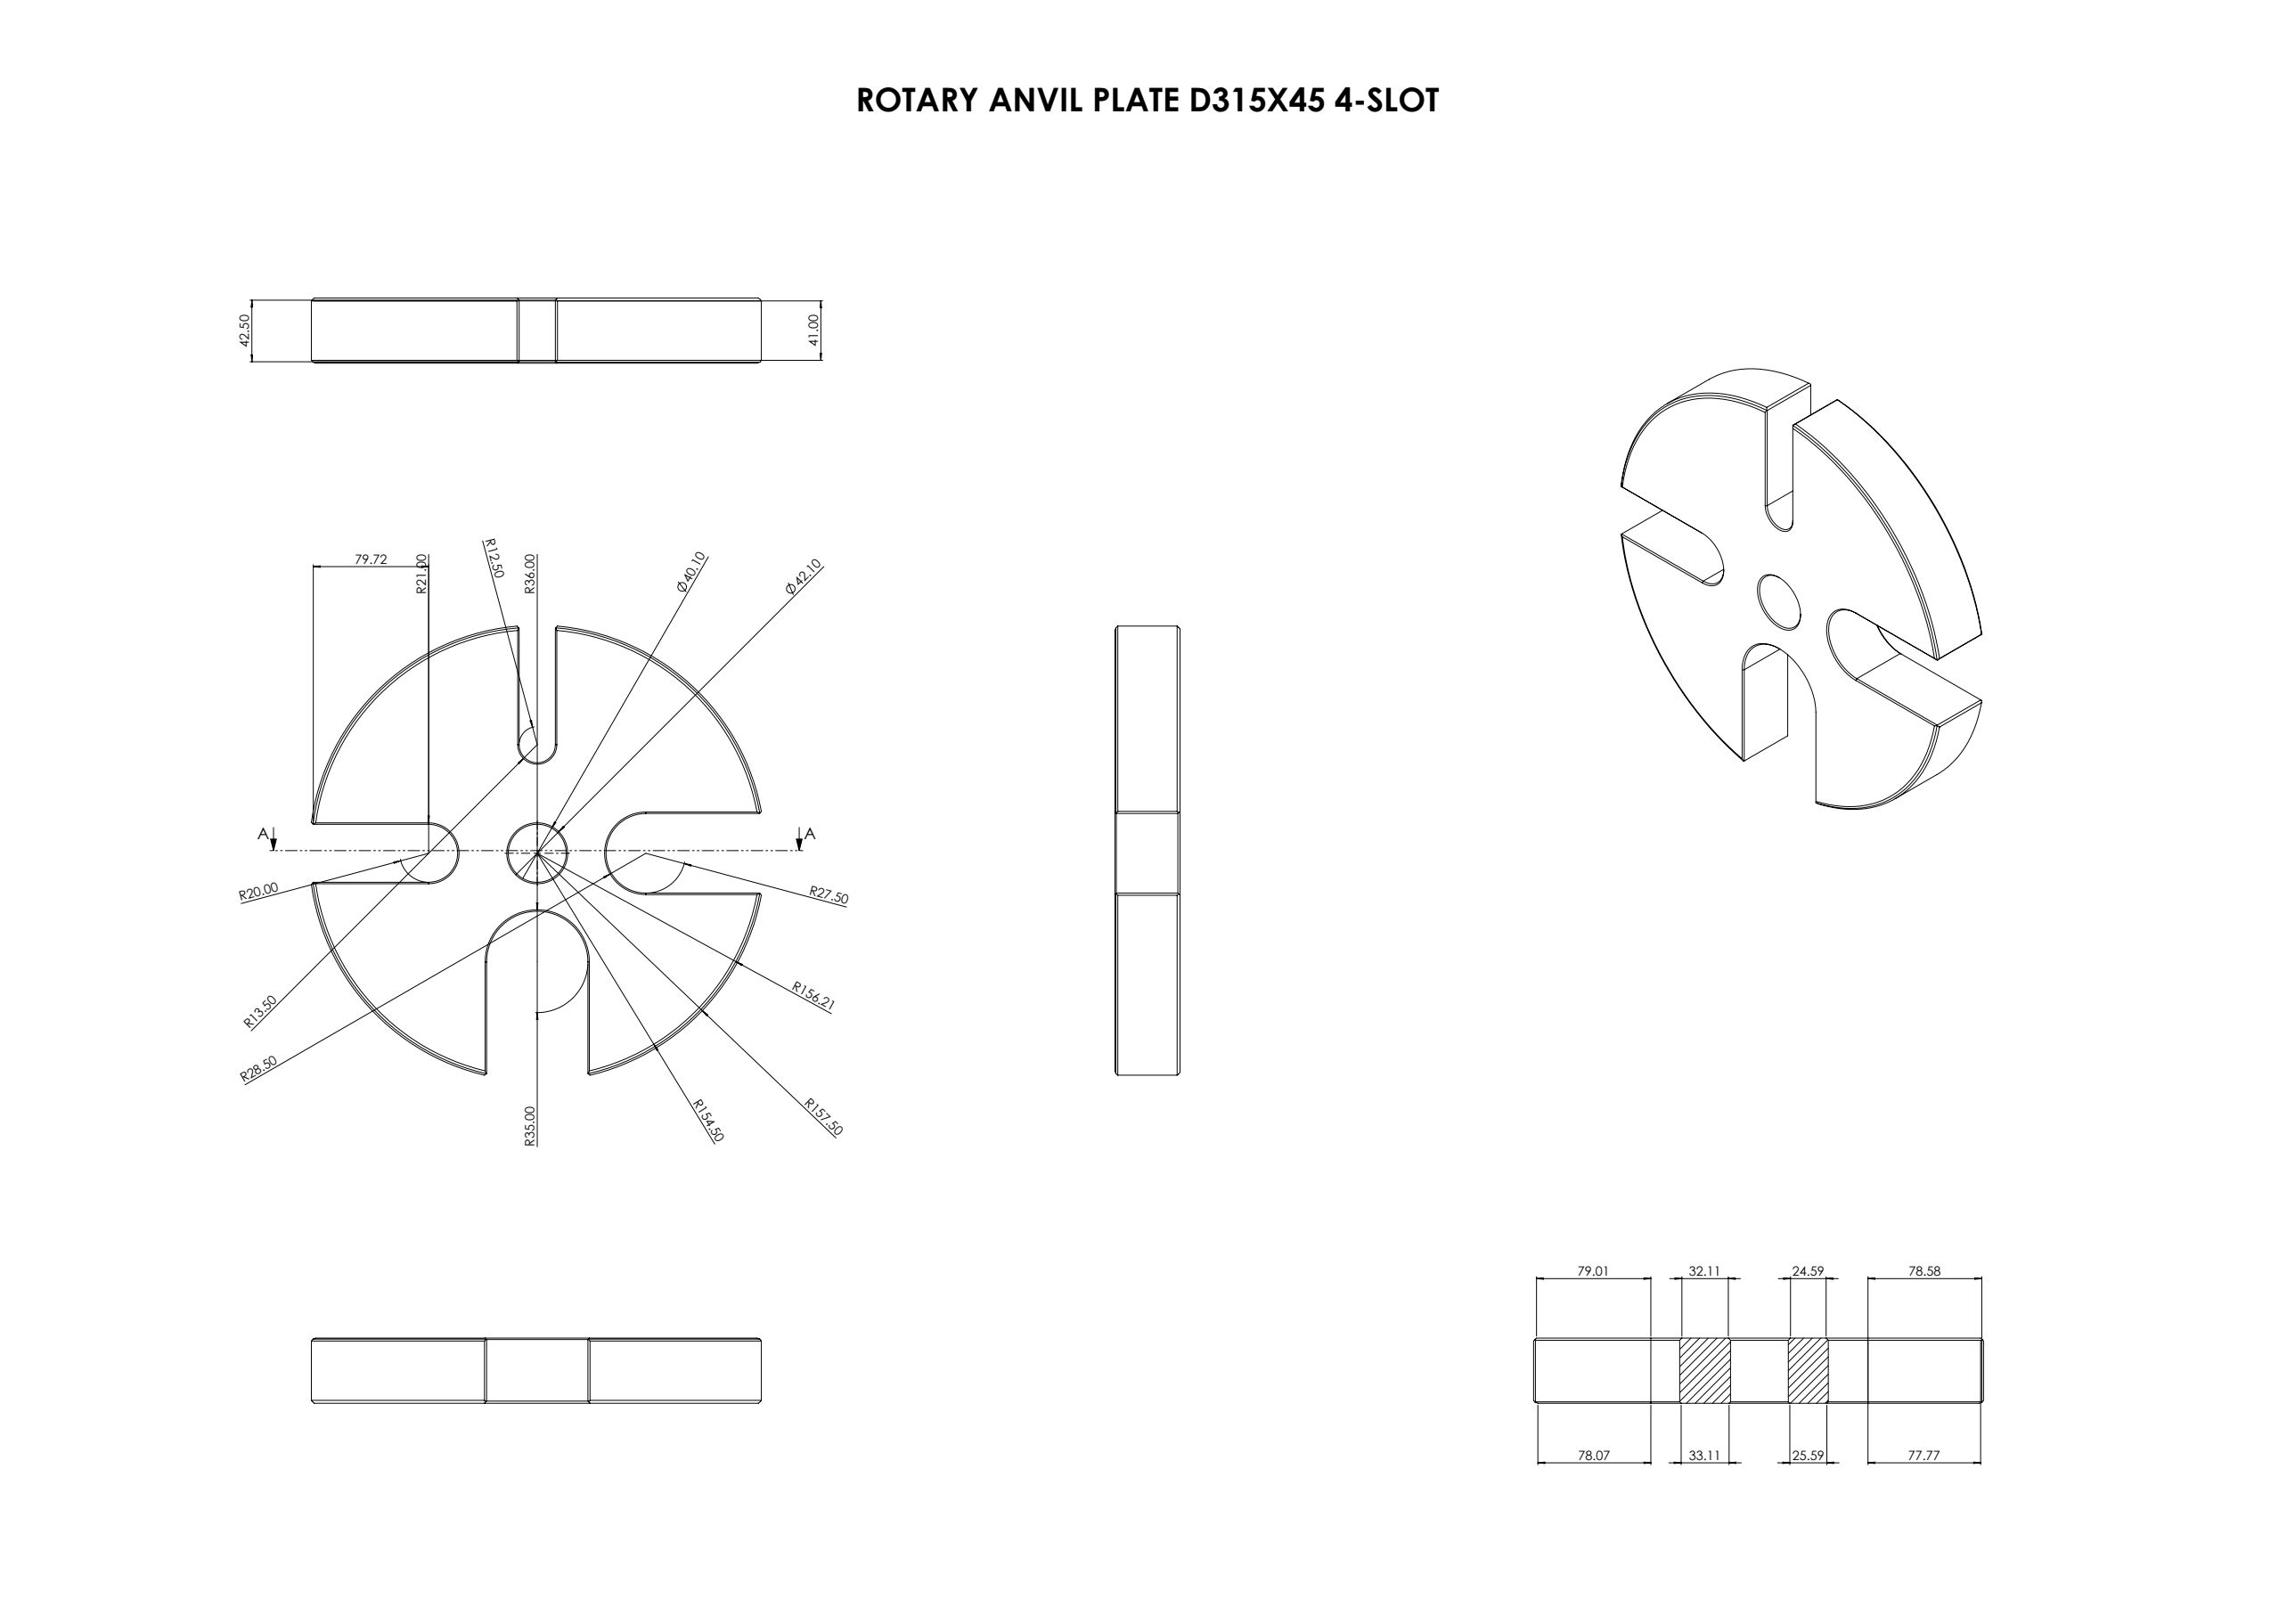
ISO-10303-21;
HEADER;
/* Generated by software containing ST-Developer
 * from STEP Tools, Inc. (www.steptools.com) 
 */

FILE_DESCRIPTION(
/* description */ (''),
/* implementation_level */ '2;1');

FILE_NAME(
/* name */ '08_Rotary_Anvil_Plate_D315x45_4-Slot.step',
/* time_stamp */ '2026-10-19T23:58:09-07:00',
/* author */ (''),
/* organization */ (''),
/* preprocessor_version */ 'ST-DEVELOPER v20.2',
/* originating_system */ 'Autodesk Translation Framework v15.15.0.0',
/* authorisation */ '');

FILE_SCHEMA (('AP203_CONFIGURATION_CONTROLLED_3D_DESIGN_OF_MECHANICAL_PARTS_AND_ASSEMBLIES_MIM_LF { 1 0 10303 203 3 1 4 }',
'AUTOMOTIVE_DESIGN { 1 0 10303 214 3 1 1 }','INTEGRATED_CNC_SCHEMA','MODEL_BASED_INTEGRATED_MANUFACTURING_SCHEMA',
'PROCESS_PLANNING_SCHEMA','AP242_MANAGED_MODEL_BASED_3D_ENGINEERING_MIM_LF { 1 0 10303 442 3 1 4 }'));
ENDSEC;

DATA;
#10=MECHANICAL_DESIGN_GEOMETRIC_PRESENTATION_REPRESENTATION('',(#409),#70757);
#171=(
BOUNDED_CURVE()
B_SPLINE_CURVE(2,(#43625,#43626,#43627),.UNSPECIFIED.,.F.,.F.)
B_SPLINE_CURVE_WITH_KNOTS((3,3),(0.00762589341662222,0.217939135937014),
 .UNSPECIFIED.)
CURVE()
GEOMETRIC_REPRESENTATION_ITEM()
RATIONAL_B_SPLINE_CURVE((1.00000105618797,1.00001509230994,1.))
REPRESENTATION_ITEM('')
);
#172=(
BOUNDED_CURVE()
B_SPLINE_CURVE(2,(#43631,#43632,#43633),.UNSPECIFIED.,.F.,.F.)
B_SPLINE_CURVE_WITH_KNOTS((3,3),(0.,0.167475634560782),.UNSPECIFIED.)
CURVE()
GEOMETRIC_REPRESENTATION_ITEM()
RATIONAL_B_SPLINE_CURVE((1.,1.00001872457605,1.00001886903166))
REPRESENTATION_ITEM('')
);
#173=(
BOUNDED_CURVE()
B_SPLINE_CURVE(2,(#43647,#43648,#43649),.UNSPECIFIED.,.F.,.F.)
B_SPLINE_CURVE_WITH_KNOTS((3,3),(0.137287012047938,0.14598329580768),
 .UNSPECIFIED.)
CURVE()
GEOMETRIC_REPRESENTATION_ITEM()
RATIONAL_B_SPLINE_CURVE((1.,1.,1.))
REPRESENTATION_ITEM('')
);
#174=(
BOUNDED_CURVE()
B_SPLINE_CURVE(2,(#43653,#43654,#43655),.UNSPECIFIED.,.F.,.F.)
B_SPLINE_CURVE_WITH_KNOTS((3,3),(7.75867498909367,7.76962220124035),
 .UNSPECIFIED.)
CURVE()
GEOMETRIC_REPRESENTATION_ITEM()
RATIONAL_B_SPLINE_CURVE((1.,1.,1.))
REPRESENTATION_ITEM('')
);
#175=(
BOUNDED_CURVE()
B_SPLINE_CURVE(2,(#43656,#43657,#43658),.UNSPECIFIED.,.F.,.F.)
B_SPLINE_CURVE_WITH_KNOTS((3,3),(0.,0.20316916463777),.UNSPECIFIED.)
CURVE()
GEOMETRIC_REPRESENTATION_ITEM()
RATIONAL_B_SPLINE_CURVE((1.,1.00001376388279,1.00000116347276))
REPRESENTATION_ITEM('')
);
#176=(
BOUNDED_CURVE()
B_SPLINE_CURVE(2,(#43673,#43674,#43675),.UNSPECIFIED.,.F.,.F.)
B_SPLINE_CURVE_WITH_KNOTS((3,3),(0.170079793729576,0.3375554282914),
 .UNSPECIFIED.)
CURVE()
GEOMETRIC_REPRESENTATION_ITEM()
RATIONAL_B_SPLINE_CURVE((1.00001886905196,1.00001872459619,1.))
REPRESENTATION_ITEM('')
);
#177=(
BOUNDED_CURVE()
B_SPLINE_CURVE(2,(#43679,#43680,#43681),.UNSPECIFIED.,.F.,.F.)
B_SPLINE_CURVE_WITH_KNOTS((3,3),(0.,0.210313242519936),.UNSPECIFIED.)
CURVE()
GEOMETRIC_REPRESENTATION_ITEM()
RATIONAL_B_SPLINE_CURVE((1.,1.00001509226017,1.00000105618449))
REPRESENTATION_ITEM('')
);
#178=(
BOUNDED_CURVE()
B_SPLINE_CURVE(2,(#43694,#43695,#43696),.UNSPECIFIED.,.F.,.F.)
B_SPLINE_CURVE_WITH_KNOTS((3,3),(0.,0.17930472101048),.UNSPECIFIED.)
CURVE()
GEOMETRIC_REPRESENTATION_ITEM()
RATIONAL_B_SPLINE_CURVE((1.,1.,1.))
REPRESENTATION_ITEM('')
);
#179=(
BOUNDED_CURVE()
B_SPLINE_CURVE(2,(#43703,#43704,#43705),.UNSPECIFIED.,.F.,.F.)
B_SPLINE_CURVE_WITH_KNOTS((3,3),(7.54305180428147,7.55174808804129),
 .UNSPECIFIED.)
CURVE()
GEOMETRIC_REPRESENTATION_ITEM()
RATIONAL_B_SPLINE_CURVE((1.,1.,1.))
REPRESENTATION_ITEM('')
);
#180=(
BOUNDED_CURVE()
B_SPLINE_CURVE(2,(#43722,#43723,#43724),.UNSPECIFIED.,.F.,.F.)
B_SPLINE_CURVE_WITH_KNOTS((3,3),(0.177416517606212,0.356721238616782),
 .UNSPECIFIED.)
CURVE()
GEOMETRIC_REPRESENTATION_ITEM()
RATIONAL_B_SPLINE_CURVE((1.,1.,1.))
REPRESENTATION_ITEM('')
);
#181=(
BOUNDED_CURVE()
B_SPLINE_CURVE(2,(#43757,#43758,#43759),.UNSPECIFIED.,.F.,.F.)
B_SPLINE_CURVE_WITH_KNOTS((3,3),(0.166982558562854,0.32848249154248),
 .UNSPECIFIED.)
CURVE()
GEOMETRIC_REPRESENTATION_ITEM()
RATIONAL_B_SPLINE_CURVE((1.00001732315097,1.00001703876093,1.))
REPRESENTATION_ITEM('')
);
#182=(
BOUNDED_CURVE()
B_SPLINE_CURVE(2,(#43760,#43761,#43762),.UNSPECIFIED.,.F.,.F.)
B_SPLINE_CURVE_WITH_KNOTS((3,3),(0.,0.188171618307079),.UNSPECIFIED.)
CURVE()
GEOMETRIC_REPRESENTATION_ITEM()
RATIONAL_B_SPLINE_CURVE((1.,1.,1.))
REPRESENTATION_ITEM('')
);
#183=(
BOUNDED_CURVE()
B_SPLINE_CURVE(2,(#43766,#43767,#43768),.UNSPECIFIED.,.F.,.F.)
B_SPLINE_CURVE_WITH_KNOTS((3,3),(0.00896598248719952,0.212135147124771),
 .UNSPECIFIED.)
CURVE()
GEOMETRIC_REPRESENTATION_ITEM()
RATIONAL_B_SPLINE_CURVE((1.00000116347024,1.00001376385308,1.))
REPRESENTATION_ITEM('')
);
#184=(
BOUNDED_CURVE()
B_SPLINE_CURVE(2,(#43772,#43773,#43774),.UNSPECIFIED.,.F.,.F.)
B_SPLINE_CURVE_WITH_KNOTS((3,3),(0.,0.161499932979635),.UNSPECIFIED.)
CURVE()
GEOMETRIC_REPRESENTATION_ITEM()
RATIONAL_B_SPLINE_CURVE((1.,1.00001703876093,1.00001732315097))
REPRESENTATION_ITEM('')
);
#185=(
BOUNDED_CURVE()
B_SPLINE_CURVE(2,(#43792,#43793,#43794),.UNSPECIFIED.,.F.,.F.)
B_SPLINE_CURVE_WITH_KNOTS((3,3),(0.143033593949376,0.153980806095915),
 .UNSPECIFIED.)
CURVE()
GEOMETRIC_REPRESENTATION_ITEM()
RATIONAL_B_SPLINE_CURVE((1.,1.,1.))
REPRESENTATION_ITEM('')
);
#186=(
BOUNDED_CURVE()
B_SPLINE_CURVE(2,(#43800,#43801,#43802),.UNSPECIFIED.,.F.,.F.)
B_SPLINE_CURVE_WITH_KNOTS((3,3),(0.18255185197649,0.370723470283569),
 .UNSPECIFIED.)
CURVE()
GEOMETRIC_REPRESENTATION_ITEM()
RATIONAL_B_SPLINE_CURVE((1.,1.,1.))
REPRESENTATION_ITEM('')
);
#187=(
BOUNDED_CURVE()
B_SPLINE_CURVE(2,(#43820,#43821,#43822),.UNSPECIFIED.,.F.,.F.)
B_SPLINE_CURVE_WITH_KNOTS((3,3),(0.166073953914202,0.324403911055146),
 .UNSPECIFIED.)
CURVE()
GEOMETRIC_REPRESENTATION_ITEM()
RATIONAL_B_SPLINE_CURVE((1.00001663891698,1.00001625098222,1.))
REPRESENTATION_ITEM('')
);
#188=(
BOUNDED_CURVE()
B_SPLINE_CURVE(2,(#43823,#43824,#43825),.UNSPECIFIED.,.F.,.F.)
B_SPLINE_CURVE_WITH_KNOTS((3,3),(0.,0.193708051007078),.UNSPECIFIED.)
CURVE()
GEOMETRIC_REPRESENTATION_ITEM()
RATIONAL_B_SPLINE_CURVE((1.,1.,1.))
REPRESENTATION_ITEM('')
);
#189=(
BOUNDED_CURVE()
B_SPLINE_CURVE(2,(#43843,#43844,#43845),.UNSPECIFIED.,.F.,.F.)
B_SPLINE_CURVE_WITH_KNOTS((3,3),(0.00815575297236999,0.214933042676883),
 .UNSPECIFIED.)
CURVE()
GEOMETRIC_REPRESENTATION_ITEM()
RATIONAL_B_SPLINE_CURVE((1.00000109358995,1.00001440998863,1.))
REPRESENTATION_ITEM('')
);
#190=(
BOUNDED_CURVE()
B_SPLINE_CURVE(2,(#43849,#43850,#43851),.UNSPECIFIED.,.F.,.F.)
B_SPLINE_CURVE_WITH_KNOTS((3,3),(0.,0.164543974719834),.UNSPECIFIED.)
CURVE()
GEOMETRIC_REPRESENTATION_ITEM()
RATIONAL_B_SPLINE_CURVE((1.,1.00001786148183,1.00001806362432))
REPRESENTATION_ITEM('')
);
#191=(
BOUNDED_CURVE()
B_SPLINE_CURVE(2,(#43869,#43870,#43871),.UNSPECIFIED.,.F.,.F.)
B_SPLINE_CURVE_WITH_KNOTS((3,3),(0.140031413282733,0.149652192224334),
 .UNSPECIFIED.)
CURVE()
GEOMETRIC_REPRESENTATION_ITEM()
RATIONAL_B_SPLINE_CURVE((1.,1.,1.))
REPRESENTATION_ITEM('')
);
#192=(
BOUNDED_CURVE()
B_SPLINE_CURVE(2,(#43877,#43878,#43879),.UNSPECIFIED.,.F.,.F.)
B_SPLINE_CURVE_WITH_KNOTS((3,3),(0.180004690478429,0.363403446267975),
 .UNSPECIFIED.)
CURVE()
GEOMETRIC_REPRESENTATION_ITEM()
RATIONAL_B_SPLINE_CURVE((1.,1.,1.))
REPRESENTATION_ITEM('')
);
#193=(
BOUNDED_CURVE()
B_SPLINE_CURVE(2,(#43884,#43885,#43886),.UNSPECIFIED.,.F.,.F.)
B_SPLINE_CURVE_WITH_KNOTS((3,3),(0.168310970500792,0.332854945221182),
 .UNSPECIFIED.)
CURVE()
GEOMETRIC_REPRESENTATION_ITEM()
RATIONAL_B_SPLINE_CURVE((1.00001806363053,1.00001786148798,1.))
REPRESENTATION_ITEM('')
);
#194=(
BOUNDED_CURVE()
B_SPLINE_CURVE(2,(#43890,#43891,#43892),.UNSPECIFIED.,.F.,.F.)
B_SPLINE_CURVE_WITH_KNOTS((3,3),(0.,0.206777289704965),.UNSPECIFIED.)
CURVE()
GEOMETRIC_REPRESENTATION_ITEM()
RATIONAL_B_SPLINE_CURVE((1.,1.00001441002009,1.00000109359234))
REPRESENTATION_ITEM('')
);
#195=(
BOUNDED_CURVE()
B_SPLINE_CURVE(2,(#43905,#43906,#43907),.UNSPECIFIED.,.F.,.F.)
B_SPLINE_CURVE_WITH_KNOTS((3,3),(0.,0.183398755789119),.UNSPECIFIED.)
CURVE()
GEOMETRIC_REPRESENTATION_ITEM()
RATIONAL_B_SPLINE_CURVE((1.,1.,1.))
REPRESENTATION_ITEM('')
);
#196=(
BOUNDED_CURVE()
B_SPLINE_CURVE(2,(#43909,#43910,#43911),.UNSPECIFIED.,.F.,.F.)
B_SPLINE_CURVE_WITH_KNOTS((3,3),(0.185074227573043,0.378782278580072),
 .UNSPECIFIED.)
CURVE()
GEOMETRIC_REPRESENTATION_ITEM()
RATIONAL_B_SPLINE_CURVE((1.,1.,1.))
REPRESENTATION_ITEM('')
);
#197=(
BOUNDED_CURVE()
B_SPLINE_CURVE(2,(#43912,#43913,#43914),.UNSPECIFIED.,.F.,.F.)
B_SPLINE_CURVE_WITH_KNOTS((3,3),(0.,0.158329957141101),.UNSPECIFIED.)
CURVE()
GEOMETRIC_REPRESENTATION_ITEM()
RATIONAL_B_SPLINE_CURVE((1.,1.00001625097861,1.00001663891328))
REPRESENTATION_ITEM('')
);
#198=(
BOUNDED_CURVE()
B_SPLINE_CURVE(2,(#43929,#43930,#43931),.UNSPECIFIED.,.F.,.F.)
B_SPLINE_CURVE_WITH_KNOTS((3,3),(0.0100528190707853,0.209523932952566),
 .UNSPECIFIED.)
CURVE()
GEOMETRIC_REPRESENTATION_ITEM()
RATIONAL_B_SPLINE_CURVE((1.00000126177961,1.00001314919847,1.))
REPRESENTATION_ITEM('')
);
#199=(
BOUNDED_CURVE()
B_SPLINE_CURVE(2,(#43949,#43950,#43951),.UNSPECIFIED.,.F.,.F.)
B_SPLINE_CURVE_WITH_KNOTS((3,3),(0.146334104657409,0.159049105721225),
 .UNSPECIFIED.)
CURVE()
GEOMETRIC_REPRESENTATION_ITEM()
RATIONAL_B_SPLINE_CURVE((1.,1.,1.))
REPRESENTATION_ITEM('')
);
#200=(
BOUNDED_CURVE()
B_SPLINE_CURVE(2,(#43962,#43963,#43964),.UNSPECIFIED.,.F.,.F.)
B_SPLINE_CURVE_WITH_KNOTS((3,3),(0.,0.199471113881606),.UNSPECIFIED.)
CURVE()
GEOMETRIC_REPRESENTATION_ITEM()
RATIONAL_B_SPLINE_CURVE((1.,1.00001314920547,1.00000126178028))
REPRESENTATION_ITEM('')
);
#201=(
BOUNDED_CURVE()
B_SPLINE_CURVE(2,(#44023,#44024,#44025),.UNSPECIFIED.,.F.,.F.)
B_SPLINE_CURVE_WITH_KNOTS((3,3),(7.87870547859755,7.89142047966152),
 .UNSPECIFIED.)
CURVE()
GEOMETRIC_REPRESENTATION_ITEM()
RATIONAL_B_SPLINE_CURVE((1.,1.,1.))
REPRESENTATION_ITEM('')
);
#202=(
BOUNDED_CURVE()
B_SPLINE_CURVE(2,(#44035,#44036,#44037),.UNSPECIFIED.,.F.,.F.)
B_SPLINE_CURVE_WITH_KNOTS((3,3),(7.6471088967316,7.6567296756733),
 .UNSPECIFIED.)
CURVE()
GEOMETRIC_REPRESENTATION_ITEM()
RATIONAL_B_SPLINE_CURVE((1.,1.,1.))
REPRESENTATION_ITEM('')
);
#379=SHAPE_REPRESENTATION_RELATIONSHIP('SRR','None',#70820,#394);
#394=ADVANCED_BREP_SHAPE_REPRESENTATION('',(#469),#70744);
#409=STYLED_ITEM('',(#71033),#469);
#469=MANIFOLD_SOLID_BREP('Anvil',#26874);
#587=CYLINDRICAL_SURFACE('',#27285,15.75);
#588=CYLINDRICAL_SURFACE('',#27319,2.75);
#589=CYLINDRICAL_SURFACE('',#27324,2.005);
#590=CYLINDRICAL_SURFACE('',#27331,15.75);
#591=CYLINDRICAL_SURFACE('',#27338,2.);
#592=CYLINDRICAL_SURFACE('',#27346,15.75);
#593=CYLINDRICAL_SURFACE('',#27351,3.5);
#594=CYLINDRICAL_SURFACE('',#27382,1.25);
#595=CYLINDRICAL_SURFACE('',#27386,15.75);
#850=FACE_BOUND('',#4238,.T.);
#851=FACE_BOUND('',#4287,.T.);
#1094=B_SPLINE_CURVE_WITH_KNOTS('',3,(#43666,#43667,#43668,#43669),
 .UNSPECIFIED.,.F.,.F.,(4,4),(0.,0.203579345120206),.UNSPECIFIED.);
#1095=B_SPLINE_CURVE_WITH_KNOTS('',3,(#43707,#43708,#43709,#43710),
 .UNSPECIFIED.,.F.,.F.,(4,4),(0.,0.203579415270987),.UNSPECIFIED.);
#1096=B_SPLINE_CURVE_WITH_KNOTS('',3,(#43788,#43789,#43790,#43791),
 .UNSPECIFIED.,.F.,.F.,(4,4),(0.,0.211711806319391),.UNSPECIFIED.);
#1097=B_SPLINE_CURVE_WITH_KNOTS('',3,(#43865,#43866,#43867,#43868),
 .UNSPECIFIED.,.F.,.F.,(4,4),(0.,0.207414265317584),.UNSPECIFIED.);
#1098=B_SPLINE_CURVE_WITH_KNOTS('',3,(#43945,#43946,#43947,#43948),
 .UNSPECIFIED.,.F.,.F.,(4,4),(0.,0.21653079565574),.UNSPECIFIED.);
#1099=B_SPLINE_CURVE_WITH_KNOTS('',3,(#43992,#43993,#43994,#43995),
 .UNSPECIFIED.,.F.,.F.,(4,4),(0.,0.207414336599568),.UNSPECIFIED.);
#1100=B_SPLINE_CURVE_WITH_KNOTS('',3,(#43999,#44000,#44001,#44002),
 .UNSPECIFIED.,.F.,.F.,(4,4),(0.,0.211711879270631),.UNSPECIFIED.);
#1101=B_SPLINE_CURVE_WITH_KNOTS('',3,(#44008,#44009,#44010,#44011),
 .UNSPECIFIED.,.F.,.F.,(4,4),(0.,0.216530870858263),.UNSPECIFIED.);
#1727=PLANE('',#27284);
#1728=PLANE('',#27290);
#1729=PLANE('',#27291);
#1730=PLANE('',#27292);
#1731=PLANE('',#27293);
#1732=PLANE('',#27294);
#1733=PLANE('',#27298);
#1734=PLANE('',#27299);
#1735=PLANE('',#27309);
#1736=PLANE('',#27310);
#1737=PLANE('',#27311);
#1738=PLANE('',#27312);
#1739=PLANE('',#27313);
#1740=PLANE('',#27314);
#1741=PLANE('',#27321);
#1742=PLANE('',#27326);
#1743=PLANE('',#27327);
#1744=PLANE('',#27328);
#1745=PLANE('',#27329);
#1746=PLANE('',#27330);
#1747=PLANE('',#27335);
#1748=PLANE('',#27340);
#1749=PLANE('',#27341);
#1750=PLANE('',#27342);
#1751=PLANE('',#27343);
#1752=PLANE('',#27344);
#1753=PLANE('',#27345);
#1754=PLANE('',#27348);
#1755=PLANE('',#27353);
#1756=PLANE('',#27367);
#1757=PLANE('',#27370);
#1758=PLANE('',#27376);
#1759=PLANE('',#27379);
#1760=PLANE('',#27383);
#2733=FACE_OUTER_BOUND('',#4227,.T.);
#2734=FACE_OUTER_BOUND('',#4228,.T.);
#2735=FACE_OUTER_BOUND('',#4229,.T.);
#2736=FACE_OUTER_BOUND('',#4230,.T.);
#2737=FACE_OUTER_BOUND('',#4231,.T.);
#2738=FACE_OUTER_BOUND('',#4232,.T.);
#2739=FACE_OUTER_BOUND('',#4233,.T.);
#2740=FACE_OUTER_BOUND('',#4234,.T.);
#2741=FACE_OUTER_BOUND('',#4235,.T.);
#2742=FACE_OUTER_BOUND('',#4236,.T.);
#2743=FACE_OUTER_BOUND('',#4237,.T.);
#2744=FACE_OUTER_BOUND('',#4239,.T.);
#2745=FACE_OUTER_BOUND('',#4240,.T.);
#2746=FACE_OUTER_BOUND('',#4241,.T.);
#2747=FACE_OUTER_BOUND('',#4242,.T.);
#2748=FACE_OUTER_BOUND('',#4243,.T.);
#2749=FACE_OUTER_BOUND('',#4244,.T.);
#2750=FACE_OUTER_BOUND('',#4245,.T.);
#2751=FACE_OUTER_BOUND('',#4246,.T.);
#2752=FACE_OUTER_BOUND('',#4247,.T.);
#2753=FACE_OUTER_BOUND('',#4248,.T.);
#2754=FACE_OUTER_BOUND('',#4249,.T.);
#2755=FACE_OUTER_BOUND('',#4250,.T.);
#2756=FACE_OUTER_BOUND('',#4251,.T.);
#2757=FACE_OUTER_BOUND('',#4252,.T.);
#2758=FACE_OUTER_BOUND('',#4253,.T.);
#2759=FACE_OUTER_BOUND('',#4254,.T.);
#2760=FACE_OUTER_BOUND('',#4255,.T.);
#2761=FACE_OUTER_BOUND('',#4256,.T.);
#2762=FACE_OUTER_BOUND('',#4257,.T.);
#2763=FACE_OUTER_BOUND('',#4258,.T.);
#2764=FACE_OUTER_BOUND('',#4259,.T.);
#2765=FACE_OUTER_BOUND('',#4260,.T.);
#2766=FACE_OUTER_BOUND('',#4261,.T.);
#2767=FACE_OUTER_BOUND('',#4262,.T.);
#2768=FACE_OUTER_BOUND('',#4263,.T.);
#2769=FACE_OUTER_BOUND('',#4264,.T.);
#2770=FACE_OUTER_BOUND('',#4265,.T.);
#2771=FACE_OUTER_BOUND('',#4266,.T.);
#2772=FACE_OUTER_BOUND('',#4267,.T.);
#2773=FACE_OUTER_BOUND('',#4268,.T.);
#2774=FACE_OUTER_BOUND('',#4269,.T.);
#2775=FACE_OUTER_BOUND('',#4270,.T.);
#2776=FACE_OUTER_BOUND('',#4271,.T.);
#2777=FACE_OUTER_BOUND('',#4272,.T.);
#2778=FACE_OUTER_BOUND('',#4273,.T.);
#2779=FACE_OUTER_BOUND('',#4274,.T.);
#2780=FACE_OUTER_BOUND('',#4275,.T.);
#2781=FACE_OUTER_BOUND('',#4276,.T.);
#2782=FACE_OUTER_BOUND('',#4277,.T.);
#2783=FACE_OUTER_BOUND('',#4278,.T.);
#2784=FACE_OUTER_BOUND('',#4279,.T.);
#2785=FACE_OUTER_BOUND('',#4280,.T.);
#2786=FACE_OUTER_BOUND('',#4281,.T.);
#2787=FACE_OUTER_BOUND('',#4282,.T.);
#2788=FACE_OUTER_BOUND('',#4283,.T.);
#2789=FACE_OUTER_BOUND('',#4284,.T.);
#2790=FACE_OUTER_BOUND('',#4285,.T.);
#2791=FACE_OUTER_BOUND('',#4286,.T.);
#2792=FACE_OUTER_BOUND('',#4288,.T.);
#2793=FACE_OUTER_BOUND('',#4289,.T.);
#2794=FACE_OUTER_BOUND('',#4290,.T.);
#2795=FACE_OUTER_BOUND('',#4291,.T.);
#2796=FACE_OUTER_BOUND('',#4292,.T.);
#2797=FACE_OUTER_BOUND('',#4293,.T.);
#4227=EDGE_LOOP('',(#18404,#18405,#18406,#18407,#18408,#18409));
#4228=EDGE_LOOP('',(#18410,#18411,#18412,#18413));
#4229=EDGE_LOOP('',(#18414,#18415,#18416,#18417,#18418,#18419));
#4230=EDGE_LOOP('',(#18420,#18421,#18422,#18423,#18424,#18425));
#4231=EDGE_LOOP('',(#18426,#18427,#18428,#18429,#18430,#18431));
#4232=EDGE_LOOP('',(#18432,#18433,#18434,#18435,#18436));
#4233=EDGE_LOOP('',(#18437,#18438,#18439,#18440));
#4234=EDGE_LOOP('',(#18441,#18442,#18443,#18444,#18445,#18446));
#4235=EDGE_LOOP('',(#18447,#18448,#18449,#18450));
#4236=EDGE_LOOP('',(#18451,#18452,#18453,#18454,#18455));
#4237=EDGE_LOOP('',(#18456,#18457,#18458,#18459,#18460,#18461,#18462,#18463,
#18464,#18465,#18466,#18467,#18468,#18469,#18470,#18471));
#4238=EDGE_LOOP('',(#18472));
#4239=EDGE_LOOP('',(#18473,#18474,#18475,#18476,#18477,#18478));
#4240=EDGE_LOOP('',(#18479,#18480,#18481,#18482,#18483,#18484));
#4241=EDGE_LOOP('',(#18485,#18486,#18487,#18488,#18489,#18490));
#4242=EDGE_LOOP('',(#18491,#18492,#18493,#18494));
#4243=EDGE_LOOP('',(#18495,#18496,#18497,#18498,#18499));
#4244=EDGE_LOOP('',(#18500,#18501,#18502,#18503,#18504,#18505));
#4245=EDGE_LOOP('',(#18506,#18507,#18508,#18509,#18510));
#4246=EDGE_LOOP('',(#18511,#18512,#18513,#18514));
#4247=EDGE_LOOP('',(#18515,#18516,#18517,#18518,#18519,#18520));
#4248=EDGE_LOOP('',(#18521,#18522,#18523,#18524));
#4249=EDGE_LOOP('',(#18525,#18526,#18527,#18528));
#4250=EDGE_LOOP('',(#18529,#18530,#18531,#18532));
#4251=EDGE_LOOP('',(#18533,#18534,#18535,#18536));
#4252=EDGE_LOOP('',(#18537,#18538,#18539,#18540,#18541,#18542));
#4253=EDGE_LOOP('',(#18543,#18544,#18545,#18546,#18547,#18548));
#4254=EDGE_LOOP('',(#18549,#18550,#18551,#18552));
#4255=EDGE_LOOP('',(#18553,#18554,#18555,#18556,#18557));
#4256=EDGE_LOOP('',(#18558,#18559,#18560,#18561,#18562,#18563));
#4257=EDGE_LOOP('',(#18564,#18565,#18566,#18567));
#4258=EDGE_LOOP('',(#18568,#18569,#18570,#18571,#18572,#18573));
#4259=EDGE_LOOP('',(#18574,#18575,#18576,#18577,#18578));
#4260=EDGE_LOOP('',(#18579,#18580,#18581,#18582));
#4261=EDGE_LOOP('',(#18583,#18584,#18585,#18586));
#4262=EDGE_LOOP('',(#18587,#18588,#18589,#18590));
#4263=EDGE_LOOP('',(#18591,#18592,#18593,#18594,#18595,#18596));
#4264=EDGE_LOOP('',(#18597,#18598,#18599,#18600,#18601,#18602));
#4265=EDGE_LOOP('',(#18603,#18604,#18605,#18606));
#4266=EDGE_LOOP('',(#18607,#18608,#18609,#18610,#18611));
#4267=EDGE_LOOP('',(#18612,#18613,#18614,#18615,#18616,#18617));
#4268=EDGE_LOOP('',(#18618,#18619,#18620,#18621));
#4269=EDGE_LOOP('',(#18622,#18623,#18624,#18625,#18626));
#4270=EDGE_LOOP('',(#18627,#18628,#18629,#18630));
#4271=EDGE_LOOP('',(#18631,#18632,#18633,#18634));
#4272=EDGE_LOOP('',(#18635,#18636,#18637,#18638));
#4273=EDGE_LOOP('',(#18639,#18640,#18641,#18642));
#4274=EDGE_LOOP('',(#18643,#18644,#18645,#18646));
#4275=EDGE_LOOP('',(#18647,#18648,#18649,#18650));
#4276=EDGE_LOOP('',(#18651,#18652,#18653,#18654));
#4277=EDGE_LOOP('',(#18655,#18656,#18657,#18658));
#4278=EDGE_LOOP('',(#18659,#18660,#18661,#18662,#18663,#18664));
#4279=EDGE_LOOP('',(#18665,#18666,#18667,#18668));
#4280=EDGE_LOOP('',(#18669,#18670,#18671,#18672,#18673,#18674));
#4281=EDGE_LOOP('',(#18675,#18676,#18677,#18678));
#4282=EDGE_LOOP('',(#18679,#18680,#18681,#18682));
#4283=EDGE_LOOP('',(#18683,#18684,#18685,#18686,#18687,#18688));
#4284=EDGE_LOOP('',(#18689,#18690,#18691,#18692,#18693,#18694));
#4285=EDGE_LOOP('',(#18695,#18696,#18697,#18698,#18699,#18700));
#4286=EDGE_LOOP('',(#18701,#18702,#18703,#18704,#18705,#18706,#18707,#18708,
#18709,#18710,#18711,#18712,#18713,#18714,#18715,#18716));
#4287=EDGE_LOOP('',(#18717));
#4288=EDGE_LOOP('',(#18718,#18719,#18720,#18721));
#4289=EDGE_LOOP('',(#18722,#18723,#18724,#18725));
#4290=EDGE_LOOP('',(#18726,#18727,#18728,#18729));
#4291=EDGE_LOOP('',(#18730,#18731,#18732,#18733,#18734,#18735));
#4292=EDGE_LOOP('',(#18736,#18737,#18738,#18739));
#4293=EDGE_LOOP('',(#18740,#18741,#18742,#18743,#18744,#18745));
#5814=LINE('',#43629,#8311);
#5815=LINE('',#43635,#8312);
#5816=LINE('',#43637,#8313);
#5817=LINE('',#43638,#8314);
#5818=LINE('',#43643,#8315);
#5819=LINE('',#43661,#8316);
#5820=LINE('',#43663,#8317);
#5821=LINE('',#43665,#8318);
#5822=LINE('',#43677,#8319);
#5823=LINE('',#43683,#8320);
#5824=LINE('',#43685,#8321);
#5825=LINE('',#43686,#8322);
#5826=LINE('',#43689,#8323);
#5827=LINE('',#43691,#8324);
#5828=LINE('',#43693,#8325);
#5829=LINE('',#43699,#8326);
#5830=LINE('',#43700,#8327);
#5831=LINE('',#43712,#8328);
#5832=LINE('',#43713,#8329);
#5833=LINE('',#43717,#8330);
#5834=LINE('',#43725,#8331);
#5835=LINE('',#43726,#8332);
#5836=LINE('',#43731,#8333);
#5837=LINE('',#43735,#8334);
#5838=LINE('',#43739,#8335);
#5839=LINE('',#43743,#8336);
#5840=LINE('',#43747,#8337);
#5841=LINE('',#43751,#8338);
#5842=LINE('',#43770,#8339);
#5843=LINE('',#43776,#8340);
#5844=LINE('',#43778,#8341);
#5845=LINE('',#43779,#8342);
#5846=LINE('',#43782,#8343);
#5847=LINE('',#43784,#8344);
#5848=LINE('',#43786,#8345);
#5849=LINE('',#43797,#8346);
#5850=LINE('',#43798,#8347);
#5851=LINE('',#43803,#8348);
#5852=LINE('',#43806,#8349);
#5853=LINE('',#43808,#8350);
#5854=LINE('',#43809,#8351);
#5855=LINE('',#43812,#8352);
#5856=LINE('',#43813,#8353);
#5857=LINE('',#43828,#8354);
#5858=LINE('',#43831,#8355);
#5859=LINE('',#43834,#8356);
#5860=LINE('',#43839,#8357);
#5861=LINE('',#43847,#8358);
#5862=LINE('',#43853,#8359);
#5863=LINE('',#43855,#8360);
#5864=LINE('',#43856,#8361);
#5865=LINE('',#43859,#8362);
#5866=LINE('',#43861,#8363);
#5867=LINE('',#43863,#8364);
#5868=LINE('',#43874,#8365);
#5869=LINE('',#43875,#8366);
#5870=LINE('',#43880,#8367);
#5871=LINE('',#43888,#8368);
#5872=LINE('',#43894,#8369);
#5873=LINE('',#43896,#8370);
#5874=LINE('',#43897,#8371);
#5875=LINE('',#43902,#8372);
#5876=LINE('',#43917,#8373);
#5877=LINE('',#43918,#8374);
#5878=LINE('',#43923,#8375);
#5879=LINE('',#43926,#8376);
#5880=LINE('',#43933,#8377);
#5881=LINE('',#43935,#8378);
#5882=LINE('',#43936,#8379);
#5883=LINE('',#43939,#8380);
#5884=LINE('',#43941,#8381);
#5885=LINE('',#43943,#8382);
#5886=LINE('',#43954,#8383);
#5887=LINE('',#43955,#8384);
#5888=LINE('',#43957,#8385);
#5889=LINE('',#43960,#8386);
#5890=LINE('',#43966,#8387);
#5891=LINE('',#43968,#8388);
#5892=LINE('',#43969,#8389);
#5893=LINE('',#43974,#8390);
#5894=LINE('',#43975,#8391);
#5895=LINE('',#43980,#8392);
#5896=LINE('',#43983,#8393);
#5897=LINE('',#44014,#8394);
#5898=LINE('',#44017,#8395);
#5899=LINE('',#44020,#8396);
#5900=LINE('',#44026,#8397);
#5901=LINE('',#44032,#8398);
#5902=LINE('',#44038,#8399);
#5903=LINE('',#44045,#8400);
#5904=LINE('',#44047,#8401);
#8311=VECTOR('',#29633,1.);
#8312=VECTOR('',#29634,1.);
#8313=VECTOR('',#29635,1.);
#8314=VECTOR('',#29636,1.);
#8315=VECTOR('',#29641,1.);
#8316=VECTOR('',#29650,1.);
#8317=VECTOR('',#29651,1.);
#8318=VECTOR('',#29652,1.);
#8319=VECTOR('',#29655,1.);
#8320=VECTOR('',#29656,1.);
#8321=VECTOR('',#29657,1.);
#8322=VECTOR('',#29658,1.);
#8323=VECTOR('',#29661,1.);
#8324=VECTOR('',#29662,1.);
#8325=VECTOR('',#29663,1.);
#8326=VECTOR('',#29666,1.);
#8327=VECTOR('',#29667,1.);
#8328=VECTOR('',#29670,1.);
#8329=VECTOR('',#29671,1.);
#8330=VECTOR('',#29674,1.);
#8331=VECTOR('',#29681,1.);
#8332=VECTOR('',#29682,1.);
#8333=VECTOR('',#29687,1.);
#8334=VECTOR('',#29690,1.);
#8335=VECTOR('',#29693,1.);
#8336=VECTOR('',#29696,1.);
#8337=VECTOR('',#29699,1.);
#8338=VECTOR('',#29702,1.);
#8339=VECTOR('',#29711,1.);
#8340=VECTOR('',#29712,1.);
#8341=VECTOR('',#29713,1.);
#8342=VECTOR('',#29714,1.);
#8343=VECTOR('',#29717,1.);
#8344=VECTOR('',#29718,1.);
#8345=VECTOR('',#29719,1.);
#8346=VECTOR('',#29722,1.);
#8347=VECTOR('',#29723,1.);
#8348=VECTOR('',#29726,1.);
#8349=VECTOR('',#29729,1.);
#8350=VECTOR('',#29730,1.);
#8351=VECTOR('',#29731,1.);
#8352=VECTOR('',#29734,1.);
#8353=VECTOR('',#29735,1.);
#8354=VECTOR('',#29746,1.);
#8355=VECTOR('',#29751,1.);
#8356=VECTOR('',#29754,2.08);
#8357=VECTOR('',#29761,2.005);
#8358=VECTOR('',#29764,1.);
#8359=VECTOR('',#29765,1.);
#8360=VECTOR('',#29766,1.);
#8361=VECTOR('',#29767,1.);
#8362=VECTOR('',#29770,1.);
#8363=VECTOR('',#29771,1.);
#8364=VECTOR('',#29772,1.);
#8365=VECTOR('',#29775,1.);
#8366=VECTOR('',#29776,1.);
#8367=VECTOR('',#29779,1.);
#8368=VECTOR('',#29782,1.);
#8369=VECTOR('',#29783,1.);
#8370=VECTOR('',#29784,1.);
#8371=VECTOR('',#29785,1.);
#8372=VECTOR('',#29790,1.);
#8373=VECTOR('',#29797,1.);
#8374=VECTOR('',#29798,1.);
#8375=VECTOR('',#29805,1.);
#8376=VECTOR('',#29810,1.);
#8377=VECTOR('',#29813,1.);
#8378=VECTOR('',#29814,1.);
#8379=VECTOR('',#29815,1.);
#8380=VECTOR('',#29818,1.);
#8381=VECTOR('',#29819,1.);
#8382=VECTOR('',#29820,1.);
#8383=VECTOR('',#29823,1.);
#8384=VECTOR('',#29824,1.);
#8385=VECTOR('',#29827,1.);
#8386=VECTOR('',#29830,1.);
#8387=VECTOR('',#29831,1.);
#8388=VECTOR('',#29832,1.);
#8389=VECTOR('',#29833,1.);
#8390=VECTOR('',#29840,1.);
#8391=VECTOR('',#29841,1.);
#8392=VECTOR('',#29848,1.);
#8393=VECTOR('',#29853,1.);
#8394=VECTOR('',#29878,1.);
#8395=VECTOR('',#29883,1.);
#8396=VECTOR('',#29886,1.);
#8397=VECTOR('',#29891,1.);
#8398=VECTOR('',#29900,1.);
#8399=VECTOR('',#29905,1.);
#8400=VECTOR('',#29916,2.055);
#8401=VECTOR('',#29919,1.);
#10726=CIRCLE('',#27286,15.75);
#10727=CIRCLE('',#27287,15.75);
#10728=CIRCLE('',#27289,15.6207106781187);
#10729=CIRCLE('',#27296,1.4);
#10730=CIRCLE('',#27297,1.25);
#10731=CIRCLE('',#27300,15.55);
#10732=CIRCLE('',#27301,2.9);
#10733=CIRCLE('',#27302,15.55);
#10734=CIRCLE('',#27303,3.65);
#10735=CIRCLE('',#27304,15.55);
#10736=CIRCLE('',#27305,2.15);
#10737=CIRCLE('',#27306,15.55);
#10738=CIRCLE('',#27307,2.155);
#10739=CIRCLE('',#27316,2.75);
#10740=CIRCLE('',#27318,15.75);
#10741=CIRCLE('',#27320,2.75);
#10742=CIRCLE('',#27323,2.005);
#10743=CIRCLE('',#27325,2.005);
#10744=CIRCLE('',#27332,15.75);
#10745=CIRCLE('',#27333,15.75);
#10746=CIRCLE('',#27337,2.);
#10747=CIRCLE('',#27339,2.);
#10748=CIRCLE('',#27347,15.75);
#10749=CIRCLE('',#27350,3.5);
#10750=CIRCLE('',#27352,3.5);
#10751=CIRCLE('',#27355,15.45);
#10752=CIRCLE('',#27356,15.6207106781187);
#10753=CIRCLE('',#27358,15.6207106781187);
#10754=CIRCLE('',#27359,15.45);
#10755=CIRCLE('',#27361,15.45);
#10756=CIRCLE('',#27363,15.6207106781187);
#10757=CIRCLE('',#27364,15.45);
#10758=CIRCLE('',#27366,2.85);
#10759=CIRCLE('',#27369,3.6);
#10760=CIRCLE('',#27372,1.35);
#10761=CIRCLE('',#27373,1.25);
#10762=CIRCLE('',#27375,2.1);
#10763=CIRCLE('',#27380,2.105);
#10764=CIRCLE('',#27385,15.75);
#10765=CIRCLE('',#27387,15.75);
#11438=VERTEX_POINT('',#43623);
#11439=VERTEX_POINT('',#43624);
#11440=VERTEX_POINT('',#43628);
#11441=VERTEX_POINT('',#43630);
#11442=VERTEX_POINT('',#43634);
#11443=VERTEX_POINT('',#43636);
#11444=VERTEX_POINT('',#43640);
#11445=VERTEX_POINT('',#43642);
#11446=VERTEX_POINT('',#43646);
#11447=VERTEX_POINT('',#43650);
#11448=VERTEX_POINT('',#43652);
#11449=VERTEX_POINT('',#43660);
#11450=VERTEX_POINT('',#43662);
#11451=VERTEX_POINT('',#43664);
#11452=VERTEX_POINT('',#43671);
#11453=VERTEX_POINT('',#43672);
#11454=VERTEX_POINT('',#43676);
#11455=VERTEX_POINT('',#43678);
#11456=VERTEX_POINT('',#43682);
#11457=VERTEX_POINT('',#43684);
#11458=VERTEX_POINT('',#43688);
#11459=VERTEX_POINT('',#43690);
#11460=VERTEX_POINT('',#43692);
#11461=VERTEX_POINT('',#43698);
#11462=VERTEX_POINT('',#43702);
#11463=VERTEX_POINT('',#43706);
#11464=VERTEX_POINT('',#43711);
#11465=VERTEX_POINT('',#43715);
#11466=VERTEX_POINT('',#43716);
#11467=VERTEX_POINT('',#43721);
#11468=VERTEX_POINT('',#43728);
#11469=VERTEX_POINT('',#43730);
#11470=VERTEX_POINT('',#43732);
#11471=VERTEX_POINT('',#43734);
#11472=VERTEX_POINT('',#43736);
#11473=VERTEX_POINT('',#43738);
#11474=VERTEX_POINT('',#43740);
#11475=VERTEX_POINT('',#43742);
#11476=VERTEX_POINT('',#43744);
#11477=VERTEX_POINT('',#43746);
#11478=VERTEX_POINT('',#43748);
#11479=VERTEX_POINT('',#43750);
#11480=VERTEX_POINT('',#43753);
#11481=VERTEX_POINT('',#43756);
#11482=VERTEX_POINT('',#43764);
#11483=VERTEX_POINT('',#43765);
#11484=VERTEX_POINT('',#43769);
#11485=VERTEX_POINT('',#43771);
#11486=VERTEX_POINT('',#43775);
#11487=VERTEX_POINT('',#43777);
#11488=VERTEX_POINT('',#43781);
#11489=VERTEX_POINT('',#43783);
#11490=VERTEX_POINT('',#43785);
#11491=VERTEX_POINT('',#43787);
#11492=VERTEX_POINT('',#43796);
#11493=VERTEX_POINT('',#43805);
#11494=VERTEX_POINT('',#43807);
#11495=VERTEX_POINT('',#43811);
#11496=VERTEX_POINT('',#43817);
#11497=VERTEX_POINT('',#43819);
#11498=VERTEX_POINT('',#43827);
#11499=VERTEX_POINT('',#43833);
#11500=VERTEX_POINT('',#43837);
#11501=VERTEX_POINT('',#43841);
#11502=VERTEX_POINT('',#43842);
#11503=VERTEX_POINT('',#43846);
#11504=VERTEX_POINT('',#43848);
#11505=VERTEX_POINT('',#43852);
#11506=VERTEX_POINT('',#43854);
#11507=VERTEX_POINT('',#43858);
#11508=VERTEX_POINT('',#43860);
#11509=VERTEX_POINT('',#43862);
#11510=VERTEX_POINT('',#43864);
#11511=VERTEX_POINT('',#43873);
#11512=VERTEX_POINT('',#43882);
#11513=VERTEX_POINT('',#43883);
#11514=VERTEX_POINT('',#43887);
#11515=VERTEX_POINT('',#43889);
#11516=VERTEX_POINT('',#43893);
#11517=VERTEX_POINT('',#43895);
#11518=VERTEX_POINT('',#43899);
#11519=VERTEX_POINT('',#43901);
#11520=VERTEX_POINT('',#43908);
#11521=VERTEX_POINT('',#43916);
#11522=VERTEX_POINT('',#43922);
#11523=VERTEX_POINT('',#43928);
#11524=VERTEX_POINT('',#43932);
#11525=VERTEX_POINT('',#43934);
#11526=VERTEX_POINT('',#43938);
#11527=VERTEX_POINT('',#43940);
#11528=VERTEX_POINT('',#43942);
#11529=VERTEX_POINT('',#43944);
#11530=VERTEX_POINT('',#43953);
#11531=VERTEX_POINT('',#43959);
#11532=VERTEX_POINT('',#43961);
#11533=VERTEX_POINT('',#43965);
#11534=VERTEX_POINT('',#43967);
#11535=VERTEX_POINT('',#43973);
#11536=VERTEX_POINT('',#43979);
#11537=VERTEX_POINT('',#43988);
#11538=VERTEX_POINT('',#43990);
#11539=VERTEX_POINT('',#43997);
#11540=VERTEX_POINT('',#44004);
#11541=VERTEX_POINT('',#44006);
#11542=VERTEX_POINT('',#44013);
#11543=VERTEX_POINT('',#44019);
#11544=VERTEX_POINT('',#44031);
#11545=VERTEX_POINT('',#44042);
#14055=EDGE_CURVE('',#11438,#11439,#171,.T.);
#14056=EDGE_CURVE('',#11439,#11440,#5814,.T.);
#14057=EDGE_CURVE('',#11440,#11441,#172,.T.);
#14058=EDGE_CURVE('',#11441,#11442,#5815,.T.);
#14059=EDGE_CURVE('',#11442,#11443,#5816,.T.);
#14060=EDGE_CURVE('',#11443,#11438,#5817,.T.);
#14061=EDGE_CURVE('',#11444,#11439,#10726,.T.);
#14062=EDGE_CURVE('',#11445,#11444,#5818,.T.);
#14063=EDGE_CURVE('',#11440,#11445,#10727,.T.);
#14064=EDGE_CURVE('',#11446,#11438,#173,.T.);
#14065=EDGE_CURVE('',#11447,#11446,#10728,.T.);
#14066=EDGE_CURVE('',#11448,#11447,#174,.T.);
#14067=EDGE_CURVE('',#11444,#11448,#175,.T.);
#14068=EDGE_CURVE('',#11443,#11449,#5819,.T.);
#14069=EDGE_CURVE('',#11449,#11450,#5820,.T.);
#14070=EDGE_CURVE('',#11450,#11451,#5821,.T.);
#14071=EDGE_CURVE('',#11446,#11451,#1094,.T.);
#14072=EDGE_CURVE('',#11452,#11453,#176,.T.);
#14073=EDGE_CURVE('',#11453,#11454,#5822,.T.);
#14074=EDGE_CURVE('',#11454,#11455,#177,.T.);
#14075=EDGE_CURVE('',#11455,#11456,#5823,.T.);
#14076=EDGE_CURVE('',#11456,#11457,#5824,.T.);
#14077=EDGE_CURVE('',#11457,#11452,#5825,.T.);
#14078=EDGE_CURVE('',#11457,#11458,#5826,.T.);
#14079=EDGE_CURVE('',#11458,#11459,#5827,.T.);
#14080=EDGE_CURVE('',#11459,#11460,#5828,.T.);
#14081=EDGE_CURVE('',#11460,#11452,#178,.T.);
#14082=EDGE_CURVE('',#11461,#11456,#5829,.T.);
#14083=EDGE_CURVE('',#11461,#11458,#5830,.T.);
#14084=EDGE_CURVE('',#11455,#11462,#179,.T.);
#14085=EDGE_CURVE('',#11463,#11462,#1095,.T.);
#14086=EDGE_CURVE('',#11463,#11464,#5831,.T.);
#14087=EDGE_CURVE('',#11461,#11464,#5832,.T.);
#14088=EDGE_CURVE('',#11465,#11466,#5833,.T.);
#14089=EDGE_CURVE('',#11466,#11459,#10729,.T.);
#14090=EDGE_CURVE('',#11458,#11465,#10730,.T.);
#14091=EDGE_CURVE('',#11441,#11467,#180,.T.);
#14092=EDGE_CURVE('',#11467,#11466,#5834,.T.);
#14093=EDGE_CURVE('',#11465,#11442,#5835,.T.);
#14094=EDGE_CURVE('',#11468,#11467,#10731,.T.);
#14095=EDGE_CURVE('',#11469,#11468,#5836,.T.);
#14096=EDGE_CURVE('',#11470,#11469,#10732,.T.);
#14097=EDGE_CURVE('',#11471,#11470,#5837,.T.);
#14098=EDGE_CURVE('',#11472,#11471,#10733,.T.);
#14099=EDGE_CURVE('',#11473,#11472,#5838,.T.);
#14100=EDGE_CURVE('',#11474,#11473,#10734,.T.);
#14101=EDGE_CURVE('',#11475,#11474,#5839,.T.);
#14102=EDGE_CURVE('',#11476,#11475,#10735,.T.);
#14103=EDGE_CURVE('',#11477,#11476,#5840,.T.);
#14104=EDGE_CURVE('',#11478,#11477,#10736,.T.);
#14105=EDGE_CURVE('',#11479,#11478,#5841,.T.);
#14106=EDGE_CURVE('',#11460,#11479,#10737,.T.);
#14107=EDGE_CURVE('',#11480,#11480,#10738,.T.);
#14108=EDGE_CURVE('',#11481,#11445,#181,.T.);
#14109=EDGE_CURVE('',#11468,#11481,#182,.T.);
#14110=EDGE_CURVE('',#11482,#11483,#183,.T.);
#14111=EDGE_CURVE('',#11483,#11484,#5842,.T.);
#14112=EDGE_CURVE('',#11484,#11485,#184,.T.);
#14113=EDGE_CURVE('',#11485,#11486,#5843,.T.);
#14114=EDGE_CURVE('',#11486,#11487,#5844,.T.);
#14115=EDGE_CURVE('',#11487,#11482,#5845,.T.);
#14116=EDGE_CURVE('',#11487,#11488,#5846,.T.);
#14117=EDGE_CURVE('',#11488,#11489,#5847,.T.);
#14118=EDGE_CURVE('',#11489,#11490,#5848,.T.);
#14119=EDGE_CURVE('',#11491,#11490,#1096,.T.);
#14120=EDGE_CURVE('',#11491,#11482,#185,.T.);
#14121=EDGE_CURVE('',#11492,#11486,#5849,.T.);
#14122=EDGE_CURVE('',#11488,#11492,#5850,.T.);
#14123=EDGE_CURVE('',#11485,#11471,#186,.T.);
#14124=EDGE_CURVE('',#11492,#11470,#5851,.T.);
#14125=EDGE_CURVE('',#11448,#11493,#5852,.T.);
#14126=EDGE_CURVE('',#11493,#11494,#5853,.T.);
#14127=EDGE_CURVE('',#11494,#11481,#5854,.T.);
#14128=EDGE_CURVE('',#11494,#11495,#5855,.T.);
#14129=EDGE_CURVE('',#11495,#11469,#5856,.T.);
#14130=EDGE_CURVE('',#11495,#11492,#10739,.T.);
#14131=EDGE_CURVE('',#11484,#11496,#10740,.T.);
#14132=EDGE_CURVE('',#11497,#11496,#187,.T.);
#14133=EDGE_CURVE('',#11472,#11497,#188,.T.);
#14134=EDGE_CURVE('',#11498,#11495,#5857,.T.);
#14135=EDGE_CURVE('',#11488,#11498,#10741,.T.);
#14136=EDGE_CURVE('',#11498,#11493,#5858,.T.);
#14137=EDGE_CURVE('',#11480,#11499,#5859,.T.);
#14138=EDGE_CURVE('',#11499,#11499,#10742,.T.);
#14139=EDGE_CURVE('',#11500,#11500,#10743,.T.);
#14140=EDGE_CURVE('',#11500,#11499,#5860,.T.);
#14141=EDGE_CURVE('',#11501,#11502,#189,.T.);
#14142=EDGE_CURVE('',#11502,#11503,#5861,.T.);
#14143=EDGE_CURVE('',#11503,#11504,#190,.T.);
#14144=EDGE_CURVE('',#11504,#11505,#5862,.T.);
#14145=EDGE_CURVE('',#11505,#11506,#5863,.T.);
#14146=EDGE_CURVE('',#11506,#11501,#5864,.T.);
#14147=EDGE_CURVE('',#11506,#11507,#5865,.T.);
#14148=EDGE_CURVE('',#11507,#11508,#5866,.T.);
#14149=EDGE_CURVE('',#11508,#11509,#5867,.T.);
#14150=EDGE_CURVE('',#11510,#11509,#1097,.T.);
#14151=EDGE_CURVE('',#11510,#11501,#191,.T.);
#14152=EDGE_CURVE('',#11511,#11505,#5868,.T.);
#14153=EDGE_CURVE('',#11507,#11511,#5869,.T.);
#14154=EDGE_CURVE('',#11504,#11479,#192,.T.);
#14155=EDGE_CURVE('',#11511,#11478,#5870,.T.);
#14156=EDGE_CURVE('',#11512,#11513,#193,.T.);
#14157=EDGE_CURVE('',#11513,#11514,#5871,.T.);
#14158=EDGE_CURVE('',#11514,#11515,#194,.T.);
#14159=EDGE_CURVE('',#11515,#11516,#5872,.T.);
#14160=EDGE_CURVE('',#11516,#11517,#5873,.T.);
#14161=EDGE_CURVE('',#11517,#11512,#5874,.T.);
#14162=EDGE_CURVE('',#11518,#11513,#10744,.T.);
#14163=EDGE_CURVE('',#11519,#11518,#5875,.T.);
#14164=EDGE_CURVE('',#11514,#11519,#10745,.T.);
#14165=EDGE_CURVE('',#11476,#11512,#195,.T.);
#14166=EDGE_CURVE('',#11520,#11475,#196,.T.);
#14167=EDGE_CURVE('',#11518,#11520,#197,.T.);
#14168=EDGE_CURVE('',#11517,#11521,#5876,.T.);
#14169=EDGE_CURVE('',#11521,#11477,#5877,.T.);
#14170=EDGE_CURVE('',#11521,#11511,#10746,.T.);
#14171=EDGE_CURVE('',#11522,#11521,#5878,.T.);
#14172=EDGE_CURVE('',#11507,#11522,#10747,.T.);
#14173=EDGE_CURVE('',#11522,#11516,#5879,.T.);
#14174=EDGE_CURVE('',#11523,#11519,#198,.T.);
#14175=EDGE_CURVE('',#11520,#11524,#5880,.T.);
#14176=EDGE_CURVE('',#11524,#11525,#5881,.T.);
#14177=EDGE_CURVE('',#11525,#11523,#5882,.T.);
#14178=EDGE_CURVE('',#11525,#11526,#5883,.T.);
#14179=EDGE_CURVE('',#11526,#11527,#5884,.T.);
#14180=EDGE_CURVE('',#11527,#11528,#5885,.T.);
#14181=EDGE_CURVE('',#11529,#11528,#1098,.T.);
#14182=EDGE_CURVE('',#11529,#11523,#199,.T.);
#14183=EDGE_CURVE('',#11530,#11524,#5886,.T.);
#14184=EDGE_CURVE('',#11526,#11530,#5887,.T.);
#14185=EDGE_CURVE('',#11530,#11474,#5888,.T.);
#14186=EDGE_CURVE('',#11496,#11531,#5889,.T.);
#14187=EDGE_CURVE('',#11531,#11532,#200,.T.);
#14188=EDGE_CURVE('',#11532,#11533,#5890,.T.);
#14189=EDGE_CURVE('',#11533,#11534,#5891,.T.);
#14190=EDGE_CURVE('',#11534,#11497,#5892,.T.);
#14191=EDGE_CURVE('',#11531,#11483,#10748,.T.);
#14192=EDGE_CURVE('',#11534,#11535,#5893,.T.);
#14193=EDGE_CURVE('',#11535,#11473,#5894,.T.);
#14194=EDGE_CURVE('',#11535,#11530,#10749,.T.);
#14195=EDGE_CURVE('',#11536,#11535,#5895,.T.);
#14196=EDGE_CURVE('',#11526,#11536,#10750,.T.);
#14197=EDGE_CURVE('',#11536,#11533,#5896,.T.);
#14198=EDGE_CURVE('',#11509,#11463,#10751,.T.);
#14199=EDGE_CURVE('',#11462,#11510,#10752,.T.);
#14200=EDGE_CURVE('',#11537,#11529,#10753,.T.);
#14201=EDGE_CURVE('',#11528,#11538,#10754,.T.);
#14202=EDGE_CURVE('',#11538,#11537,#1099,.T.);
#14203=EDGE_CURVE('',#11451,#11539,#10755,.T.);
#14204=EDGE_CURVE('',#11539,#11447,#1100,.T.);
#14205=EDGE_CURVE('',#11540,#11491,#10756,.T.);
#14206=EDGE_CURVE('',#11490,#11541,#10757,.T.);
#14207=EDGE_CURVE('',#11541,#11540,#1101,.T.);
#14208=EDGE_CURVE('',#11498,#11542,#5897,.T.);
#14209=EDGE_CURVE('',#11542,#11489,#10758,.T.);
#14210=EDGE_CURVE('',#11539,#11542,#5898,.T.);
#14211=EDGE_CURVE('',#11536,#11543,#5899,.T.);
#14212=EDGE_CURVE('',#11543,#11527,#10759,.T.);
#14213=EDGE_CURVE('',#11532,#11540,#201,.T.);
#14214=EDGE_CURVE('',#11541,#11543,#5900,.T.);
#14215=EDGE_CURVE('',#11464,#11450,#10760,.T.);
#14216=EDGE_CURVE('',#11449,#11461,#10761,.T.);
#14217=EDGE_CURVE('',#11522,#11544,#5901,.T.);
#14218=EDGE_CURVE('',#11544,#11508,#10762,.T.);
#14219=EDGE_CURVE('',#11515,#11537,#202,.T.);
#14220=EDGE_CURVE('',#11538,#11544,#5902,.T.);
#14221=EDGE_CURVE('',#11545,#11545,#10763,.T.);
#14222=EDGE_CURVE('',#11545,#11500,#5903,.T.);
#14223=EDGE_CURVE('',#11449,#11465,#5904,.T.);
#14224=EDGE_CURVE('',#11454,#11502,#10764,.T.);
#14225=EDGE_CURVE('',#11503,#11453,#10765,.T.);
#18404=ORIENTED_EDGE('',*,*,#14055,.T.);
#18405=ORIENTED_EDGE('',*,*,#14056,.T.);
#18406=ORIENTED_EDGE('',*,*,#14057,.T.);
#18407=ORIENTED_EDGE('',*,*,#14058,.T.);
#18408=ORIENTED_EDGE('',*,*,#14059,.T.);
#18409=ORIENTED_EDGE('',*,*,#14060,.T.);
#18410=ORIENTED_EDGE('',*,*,#14056,.F.);
#18411=ORIENTED_EDGE('',*,*,#14061,.F.);
#18412=ORIENTED_EDGE('',*,*,#14062,.F.);
#18413=ORIENTED_EDGE('',*,*,#14063,.F.);
#18414=ORIENTED_EDGE('',*,*,#14055,.F.);
#18415=ORIENTED_EDGE('',*,*,#14064,.F.);
#18416=ORIENTED_EDGE('',*,*,#14065,.F.);
#18417=ORIENTED_EDGE('',*,*,#14066,.F.);
#18418=ORIENTED_EDGE('',*,*,#14067,.F.);
#18419=ORIENTED_EDGE('',*,*,#14061,.T.);
#18420=ORIENTED_EDGE('',*,*,#14060,.F.);
#18421=ORIENTED_EDGE('',*,*,#14068,.T.);
#18422=ORIENTED_EDGE('',*,*,#14069,.T.);
#18423=ORIENTED_EDGE('',*,*,#14070,.T.);
#18424=ORIENTED_EDGE('',*,*,#14071,.F.);
#18425=ORIENTED_EDGE('',*,*,#14064,.T.);
#18426=ORIENTED_EDGE('',*,*,#14072,.T.);
#18427=ORIENTED_EDGE('',*,*,#14073,.T.);
#18428=ORIENTED_EDGE('',*,*,#14074,.T.);
#18429=ORIENTED_EDGE('',*,*,#14075,.T.);
#18430=ORIENTED_EDGE('',*,*,#14076,.T.);
#18431=ORIENTED_EDGE('',*,*,#14077,.T.);
#18432=ORIENTED_EDGE('',*,*,#14077,.F.);
#18433=ORIENTED_EDGE('',*,*,#14078,.T.);
#18434=ORIENTED_EDGE('',*,*,#14079,.T.);
#18435=ORIENTED_EDGE('',*,*,#14080,.T.);
#18436=ORIENTED_EDGE('',*,*,#14081,.T.);
#18437=ORIENTED_EDGE('',*,*,#14076,.F.);
#18438=ORIENTED_EDGE('',*,*,#14082,.F.);
#18439=ORIENTED_EDGE('',*,*,#14083,.T.);
#18440=ORIENTED_EDGE('',*,*,#14078,.F.);
#18441=ORIENTED_EDGE('',*,*,#14075,.F.);
#18442=ORIENTED_EDGE('',*,*,#14084,.T.);
#18443=ORIENTED_EDGE('',*,*,#14085,.F.);
#18444=ORIENTED_EDGE('',*,*,#14086,.T.);
#18445=ORIENTED_EDGE('',*,*,#14087,.F.);
#18446=ORIENTED_EDGE('',*,*,#14082,.T.);
#18447=ORIENTED_EDGE('',*,*,#14088,.T.);
#18448=ORIENTED_EDGE('',*,*,#14089,.T.);
#18449=ORIENTED_EDGE('',*,*,#14079,.F.);
#18450=ORIENTED_EDGE('',*,*,#14090,.T.);
#18451=ORIENTED_EDGE('',*,*,#14058,.F.);
#18452=ORIENTED_EDGE('',*,*,#14091,.T.);
#18453=ORIENTED_EDGE('',*,*,#14092,.T.);
#18454=ORIENTED_EDGE('',*,*,#14088,.F.);
#18455=ORIENTED_EDGE('',*,*,#14093,.T.);
#18456=ORIENTED_EDGE('',*,*,#14080,.F.);
#18457=ORIENTED_EDGE('',*,*,#14089,.F.);
#18458=ORIENTED_EDGE('',*,*,#14092,.F.);
#18459=ORIENTED_EDGE('',*,*,#14094,.F.);
#18460=ORIENTED_EDGE('',*,*,#14095,.F.);
#18461=ORIENTED_EDGE('',*,*,#14096,.F.);
#18462=ORIENTED_EDGE('',*,*,#14097,.F.);
#18463=ORIENTED_EDGE('',*,*,#14098,.F.);
#18464=ORIENTED_EDGE('',*,*,#14099,.F.);
#18465=ORIENTED_EDGE('',*,*,#14100,.F.);
#18466=ORIENTED_EDGE('',*,*,#14101,.F.);
#18467=ORIENTED_EDGE('',*,*,#14102,.F.);
#18468=ORIENTED_EDGE('',*,*,#14103,.F.);
#18469=ORIENTED_EDGE('',*,*,#14104,.F.);
#18470=ORIENTED_EDGE('',*,*,#14105,.F.);
#18471=ORIENTED_EDGE('',*,*,#14106,.F.);
#18472=ORIENTED_EDGE('',*,*,#14107,.F.);
#18473=ORIENTED_EDGE('',*,*,#14057,.F.);
#18474=ORIENTED_EDGE('',*,*,#14063,.T.);
#18475=ORIENTED_EDGE('',*,*,#14108,.F.);
#18476=ORIENTED_EDGE('',*,*,#14109,.F.);
#18477=ORIENTED_EDGE('',*,*,#14094,.T.);
#18478=ORIENTED_EDGE('',*,*,#14091,.F.);
#18479=ORIENTED_EDGE('',*,*,#14110,.T.);
#18480=ORIENTED_EDGE('',*,*,#14111,.T.);
#18481=ORIENTED_EDGE('',*,*,#14112,.T.);
#18482=ORIENTED_EDGE('',*,*,#14113,.T.);
#18483=ORIENTED_EDGE('',*,*,#14114,.T.);
#18484=ORIENTED_EDGE('',*,*,#14115,.T.);
#18485=ORIENTED_EDGE('',*,*,#14115,.F.);
#18486=ORIENTED_EDGE('',*,*,#14116,.T.);
#18487=ORIENTED_EDGE('',*,*,#14117,.T.);
#18488=ORIENTED_EDGE('',*,*,#14118,.T.);
#18489=ORIENTED_EDGE('',*,*,#14119,.F.);
#18490=ORIENTED_EDGE('',*,*,#14120,.T.);
#18491=ORIENTED_EDGE('',*,*,#14114,.F.);
#18492=ORIENTED_EDGE('',*,*,#14121,.F.);
#18493=ORIENTED_EDGE('',*,*,#14122,.F.);
#18494=ORIENTED_EDGE('',*,*,#14116,.F.);
#18495=ORIENTED_EDGE('',*,*,#14113,.F.);
#18496=ORIENTED_EDGE('',*,*,#14123,.T.);
#18497=ORIENTED_EDGE('',*,*,#14097,.T.);
#18498=ORIENTED_EDGE('',*,*,#14124,.F.);
#18499=ORIENTED_EDGE('',*,*,#14121,.T.);
#18500=ORIENTED_EDGE('',*,*,#14108,.T.);
#18501=ORIENTED_EDGE('',*,*,#14062,.T.);
#18502=ORIENTED_EDGE('',*,*,#14067,.T.);
#18503=ORIENTED_EDGE('',*,*,#14125,.T.);
#18504=ORIENTED_EDGE('',*,*,#14126,.T.);
#18505=ORIENTED_EDGE('',*,*,#14127,.T.);
#18506=ORIENTED_EDGE('',*,*,#14127,.F.);
#18507=ORIENTED_EDGE('',*,*,#14128,.T.);
#18508=ORIENTED_EDGE('',*,*,#14129,.T.);
#18509=ORIENTED_EDGE('',*,*,#14095,.T.);
#18510=ORIENTED_EDGE('',*,*,#14109,.T.);
#18511=ORIENTED_EDGE('',*,*,#14124,.T.);
#18512=ORIENTED_EDGE('',*,*,#14096,.T.);
#18513=ORIENTED_EDGE('',*,*,#14129,.F.);
#18514=ORIENTED_EDGE('',*,*,#14130,.T.);
#18515=ORIENTED_EDGE('',*,*,#14112,.F.);
#18516=ORIENTED_EDGE('',*,*,#14131,.T.);
#18517=ORIENTED_EDGE('',*,*,#14132,.F.);
#18518=ORIENTED_EDGE('',*,*,#14133,.F.);
#18519=ORIENTED_EDGE('',*,*,#14098,.T.);
#18520=ORIENTED_EDGE('',*,*,#14123,.F.);
#18521=ORIENTED_EDGE('',*,*,#14130,.F.);
#18522=ORIENTED_EDGE('',*,*,#14134,.F.);
#18523=ORIENTED_EDGE('',*,*,#14135,.F.);
#18524=ORIENTED_EDGE('',*,*,#14122,.T.);
#18525=ORIENTED_EDGE('',*,*,#14126,.F.);
#18526=ORIENTED_EDGE('',*,*,#14136,.F.);
#18527=ORIENTED_EDGE('',*,*,#14134,.T.);
#18528=ORIENTED_EDGE('',*,*,#14128,.F.);
#18529=ORIENTED_EDGE('',*,*,#14107,.T.);
#18530=ORIENTED_EDGE('',*,*,#14137,.T.);
#18531=ORIENTED_EDGE('',*,*,#14138,.T.);
#18532=ORIENTED_EDGE('',*,*,#14137,.F.);
#18533=ORIENTED_EDGE('',*,*,#14139,.F.);
#18534=ORIENTED_EDGE('',*,*,#14140,.T.);
#18535=ORIENTED_EDGE('',*,*,#14138,.F.);
#18536=ORIENTED_EDGE('',*,*,#14140,.F.);
#18537=ORIENTED_EDGE('',*,*,#14141,.T.);
#18538=ORIENTED_EDGE('',*,*,#14142,.T.);
#18539=ORIENTED_EDGE('',*,*,#14143,.T.);
#18540=ORIENTED_EDGE('',*,*,#14144,.T.);
#18541=ORIENTED_EDGE('',*,*,#14145,.T.);
#18542=ORIENTED_EDGE('',*,*,#14146,.T.);
#18543=ORIENTED_EDGE('',*,*,#14146,.F.);
#18544=ORIENTED_EDGE('',*,*,#14147,.T.);
#18545=ORIENTED_EDGE('',*,*,#14148,.T.);
#18546=ORIENTED_EDGE('',*,*,#14149,.T.);
#18547=ORIENTED_EDGE('',*,*,#14150,.F.);
#18548=ORIENTED_EDGE('',*,*,#14151,.T.);
#18549=ORIENTED_EDGE('',*,*,#14145,.F.);
#18550=ORIENTED_EDGE('',*,*,#14152,.F.);
#18551=ORIENTED_EDGE('',*,*,#14153,.F.);
#18552=ORIENTED_EDGE('',*,*,#14147,.F.);
#18553=ORIENTED_EDGE('',*,*,#14144,.F.);
#18554=ORIENTED_EDGE('',*,*,#14154,.T.);
#18555=ORIENTED_EDGE('',*,*,#14105,.T.);
#18556=ORIENTED_EDGE('',*,*,#14155,.F.);
#18557=ORIENTED_EDGE('',*,*,#14152,.T.);
#18558=ORIENTED_EDGE('',*,*,#14156,.T.);
#18559=ORIENTED_EDGE('',*,*,#14157,.T.);
#18560=ORIENTED_EDGE('',*,*,#14158,.T.);
#18561=ORIENTED_EDGE('',*,*,#14159,.T.);
#18562=ORIENTED_EDGE('',*,*,#14160,.T.);
#18563=ORIENTED_EDGE('',*,*,#14161,.T.);
#18564=ORIENTED_EDGE('',*,*,#14157,.F.);
#18565=ORIENTED_EDGE('',*,*,#14162,.F.);
#18566=ORIENTED_EDGE('',*,*,#14163,.F.);
#18567=ORIENTED_EDGE('',*,*,#14164,.F.);
#18568=ORIENTED_EDGE('',*,*,#14156,.F.);
#18569=ORIENTED_EDGE('',*,*,#14165,.F.);
#18570=ORIENTED_EDGE('',*,*,#14102,.T.);
#18571=ORIENTED_EDGE('',*,*,#14166,.F.);
#18572=ORIENTED_EDGE('',*,*,#14167,.F.);
#18573=ORIENTED_EDGE('',*,*,#14162,.T.);
#18574=ORIENTED_EDGE('',*,*,#14161,.F.);
#18575=ORIENTED_EDGE('',*,*,#14168,.T.);
#18576=ORIENTED_EDGE('',*,*,#14169,.T.);
#18577=ORIENTED_EDGE('',*,*,#14103,.T.);
#18578=ORIENTED_EDGE('',*,*,#14165,.T.);
#18579=ORIENTED_EDGE('',*,*,#14155,.T.);
#18580=ORIENTED_EDGE('',*,*,#14104,.T.);
#18581=ORIENTED_EDGE('',*,*,#14169,.F.);
#18582=ORIENTED_EDGE('',*,*,#14170,.T.);
#18583=ORIENTED_EDGE('',*,*,#14170,.F.);
#18584=ORIENTED_EDGE('',*,*,#14171,.F.);
#18585=ORIENTED_EDGE('',*,*,#14172,.F.);
#18586=ORIENTED_EDGE('',*,*,#14153,.T.);
#18587=ORIENTED_EDGE('',*,*,#14160,.F.);
#18588=ORIENTED_EDGE('',*,*,#14173,.F.);
#18589=ORIENTED_EDGE('',*,*,#14171,.T.);
#18590=ORIENTED_EDGE('',*,*,#14168,.F.);
#18591=ORIENTED_EDGE('',*,*,#14174,.T.);
#18592=ORIENTED_EDGE('',*,*,#14163,.T.);
#18593=ORIENTED_EDGE('',*,*,#14167,.T.);
#18594=ORIENTED_EDGE('',*,*,#14175,.T.);
#18595=ORIENTED_EDGE('',*,*,#14176,.T.);
#18596=ORIENTED_EDGE('',*,*,#14177,.T.);
#18597=ORIENTED_EDGE('',*,*,#14177,.F.);
#18598=ORIENTED_EDGE('',*,*,#14178,.T.);
#18599=ORIENTED_EDGE('',*,*,#14179,.T.);
#18600=ORIENTED_EDGE('',*,*,#14180,.T.);
#18601=ORIENTED_EDGE('',*,*,#14181,.F.);
#18602=ORIENTED_EDGE('',*,*,#14182,.T.);
#18603=ORIENTED_EDGE('',*,*,#14176,.F.);
#18604=ORIENTED_EDGE('',*,*,#14183,.F.);
#18605=ORIENTED_EDGE('',*,*,#14184,.F.);
#18606=ORIENTED_EDGE('',*,*,#14178,.F.);
#18607=ORIENTED_EDGE('',*,*,#14175,.F.);
#18608=ORIENTED_EDGE('',*,*,#14166,.T.);
#18609=ORIENTED_EDGE('',*,*,#14101,.T.);
#18610=ORIENTED_EDGE('',*,*,#14185,.F.);
#18611=ORIENTED_EDGE('',*,*,#14183,.T.);
#18612=ORIENTED_EDGE('',*,*,#14132,.T.);
#18613=ORIENTED_EDGE('',*,*,#14186,.T.);
#18614=ORIENTED_EDGE('',*,*,#14187,.T.);
#18615=ORIENTED_EDGE('',*,*,#14188,.T.);
#18616=ORIENTED_EDGE('',*,*,#14189,.T.);
#18617=ORIENTED_EDGE('',*,*,#14190,.T.);
#18618=ORIENTED_EDGE('',*,*,#14111,.F.);
#18619=ORIENTED_EDGE('',*,*,#14191,.F.);
#18620=ORIENTED_EDGE('',*,*,#14186,.F.);
#18621=ORIENTED_EDGE('',*,*,#14131,.F.);
#18622=ORIENTED_EDGE('',*,*,#14190,.F.);
#18623=ORIENTED_EDGE('',*,*,#14192,.T.);
#18624=ORIENTED_EDGE('',*,*,#14193,.T.);
#18625=ORIENTED_EDGE('',*,*,#14099,.T.);
#18626=ORIENTED_EDGE('',*,*,#14133,.T.);
#18627=ORIENTED_EDGE('',*,*,#14185,.T.);
#18628=ORIENTED_EDGE('',*,*,#14100,.T.);
#18629=ORIENTED_EDGE('',*,*,#14193,.F.);
#18630=ORIENTED_EDGE('',*,*,#14194,.T.);
#18631=ORIENTED_EDGE('',*,*,#14194,.F.);
#18632=ORIENTED_EDGE('',*,*,#14195,.F.);
#18633=ORIENTED_EDGE('',*,*,#14196,.F.);
#18634=ORIENTED_EDGE('',*,*,#14184,.T.);
#18635=ORIENTED_EDGE('',*,*,#14189,.F.);
#18636=ORIENTED_EDGE('',*,*,#14197,.F.);
#18637=ORIENTED_EDGE('',*,*,#14195,.T.);
#18638=ORIENTED_EDGE('',*,*,#14192,.F.);
#18639=ORIENTED_EDGE('',*,*,#14198,.T.);
#18640=ORIENTED_EDGE('',*,*,#14085,.T.);
#18641=ORIENTED_EDGE('',*,*,#14199,.T.);
#18642=ORIENTED_EDGE('',*,*,#14150,.T.);
#18643=ORIENTED_EDGE('',*,*,#14200,.T.);
#18644=ORIENTED_EDGE('',*,*,#14181,.T.);
#18645=ORIENTED_EDGE('',*,*,#14201,.T.);
#18646=ORIENTED_EDGE('',*,*,#14202,.T.);
#18647=ORIENTED_EDGE('',*,*,#14203,.T.);
#18648=ORIENTED_EDGE('',*,*,#14204,.T.);
#18649=ORIENTED_EDGE('',*,*,#14065,.T.);
#18650=ORIENTED_EDGE('',*,*,#14071,.T.);
#18651=ORIENTED_EDGE('',*,*,#14205,.T.);
#18652=ORIENTED_EDGE('',*,*,#14119,.T.);
#18653=ORIENTED_EDGE('',*,*,#14206,.T.);
#18654=ORIENTED_EDGE('',*,*,#14207,.T.);
#18655=ORIENTED_EDGE('',*,*,#14208,.T.);
#18656=ORIENTED_EDGE('',*,*,#14209,.T.);
#18657=ORIENTED_EDGE('',*,*,#14117,.F.);
#18658=ORIENTED_EDGE('',*,*,#14135,.T.);
#18659=ORIENTED_EDGE('',*,*,#14125,.F.);
#18660=ORIENTED_EDGE('',*,*,#14066,.T.);
#18661=ORIENTED_EDGE('',*,*,#14204,.F.);
#18662=ORIENTED_EDGE('',*,*,#14210,.T.);
#18663=ORIENTED_EDGE('',*,*,#14208,.F.);
#18664=ORIENTED_EDGE('',*,*,#14136,.T.);
#18665=ORIENTED_EDGE('',*,*,#14211,.T.);
#18666=ORIENTED_EDGE('',*,*,#14212,.T.);
#18667=ORIENTED_EDGE('',*,*,#14179,.F.);
#18668=ORIENTED_EDGE('',*,*,#14196,.T.);
#18669=ORIENTED_EDGE('',*,*,#14188,.F.);
#18670=ORIENTED_EDGE('',*,*,#14213,.T.);
#18671=ORIENTED_EDGE('',*,*,#14207,.F.);
#18672=ORIENTED_EDGE('',*,*,#14214,.T.);
#18673=ORIENTED_EDGE('',*,*,#14211,.F.);
#18674=ORIENTED_EDGE('',*,*,#14197,.T.);
#18675=ORIENTED_EDGE('',*,*,#14087,.T.);
#18676=ORIENTED_EDGE('',*,*,#14215,.T.);
#18677=ORIENTED_EDGE('',*,*,#14069,.F.);
#18678=ORIENTED_EDGE('',*,*,#14216,.T.);
#18679=ORIENTED_EDGE('',*,*,#14217,.T.);
#18680=ORIENTED_EDGE('',*,*,#14218,.T.);
#18681=ORIENTED_EDGE('',*,*,#14148,.F.);
#18682=ORIENTED_EDGE('',*,*,#14172,.T.);
#18683=ORIENTED_EDGE('',*,*,#14159,.F.);
#18684=ORIENTED_EDGE('',*,*,#14219,.T.);
#18685=ORIENTED_EDGE('',*,*,#14202,.F.);
#18686=ORIENTED_EDGE('',*,*,#14220,.T.);
#18687=ORIENTED_EDGE('',*,*,#14217,.F.);
#18688=ORIENTED_EDGE('',*,*,#14173,.T.);
#18689=ORIENTED_EDGE('',*,*,#14110,.F.);
#18690=ORIENTED_EDGE('',*,*,#14120,.F.);
#18691=ORIENTED_EDGE('',*,*,#14205,.F.);
#18692=ORIENTED_EDGE('',*,*,#14213,.F.);
#18693=ORIENTED_EDGE('',*,*,#14187,.F.);
#18694=ORIENTED_EDGE('',*,*,#14191,.T.);
#18695=ORIENTED_EDGE('',*,*,#14158,.F.);
#18696=ORIENTED_EDGE('',*,*,#14164,.T.);
#18697=ORIENTED_EDGE('',*,*,#14174,.F.);
#18698=ORIENTED_EDGE('',*,*,#14182,.F.);
#18699=ORIENTED_EDGE('',*,*,#14200,.F.);
#18700=ORIENTED_EDGE('',*,*,#14219,.F.);
#18701=ORIENTED_EDGE('',*,*,#14206,.F.);
#18702=ORIENTED_EDGE('',*,*,#14118,.F.);
#18703=ORIENTED_EDGE('',*,*,#14209,.F.);
#18704=ORIENTED_EDGE('',*,*,#14210,.F.);
#18705=ORIENTED_EDGE('',*,*,#14203,.F.);
#18706=ORIENTED_EDGE('',*,*,#14070,.F.);
#18707=ORIENTED_EDGE('',*,*,#14215,.F.);
#18708=ORIENTED_EDGE('',*,*,#14086,.F.);
#18709=ORIENTED_EDGE('',*,*,#14198,.F.);
#18710=ORIENTED_EDGE('',*,*,#14149,.F.);
#18711=ORIENTED_EDGE('',*,*,#14218,.F.);
#18712=ORIENTED_EDGE('',*,*,#14220,.F.);
#18713=ORIENTED_EDGE('',*,*,#14201,.F.);
#18714=ORIENTED_EDGE('',*,*,#14180,.F.);
#18715=ORIENTED_EDGE('',*,*,#14212,.F.);
#18716=ORIENTED_EDGE('',*,*,#14214,.F.);
#18717=ORIENTED_EDGE('',*,*,#14221,.F.);
#18718=ORIENTED_EDGE('',*,*,#14221,.T.);
#18719=ORIENTED_EDGE('',*,*,#14222,.T.);
#18720=ORIENTED_EDGE('',*,*,#14139,.T.);
#18721=ORIENTED_EDGE('',*,*,#14222,.F.);
#18722=ORIENTED_EDGE('',*,*,#14090,.F.);
#18723=ORIENTED_EDGE('',*,*,#14083,.F.);
#18724=ORIENTED_EDGE('',*,*,#14216,.F.);
#18725=ORIENTED_EDGE('',*,*,#14223,.T.);
#18726=ORIENTED_EDGE('',*,*,#14059,.F.);
#18727=ORIENTED_EDGE('',*,*,#14093,.F.);
#18728=ORIENTED_EDGE('',*,*,#14223,.F.);
#18729=ORIENTED_EDGE('',*,*,#14068,.F.);
#18730=ORIENTED_EDGE('',*,*,#14074,.F.);
#18731=ORIENTED_EDGE('',*,*,#14224,.T.);
#18732=ORIENTED_EDGE('',*,*,#14141,.F.);
#18733=ORIENTED_EDGE('',*,*,#14151,.F.);
#18734=ORIENTED_EDGE('',*,*,#14199,.F.);
#18735=ORIENTED_EDGE('',*,*,#14084,.F.);
#18736=ORIENTED_EDGE('',*,*,#14073,.F.);
#18737=ORIENTED_EDGE('',*,*,#14225,.F.);
#18738=ORIENTED_EDGE('',*,*,#14142,.F.);
#18739=ORIENTED_EDGE('',*,*,#14224,.F.);
#18740=ORIENTED_EDGE('',*,*,#14072,.F.);
#18741=ORIENTED_EDGE('',*,*,#14081,.F.);
#18742=ORIENTED_EDGE('',*,*,#14106,.T.);
#18743=ORIENTED_EDGE('',*,*,#14154,.F.);
#18744=ORIENTED_EDGE('',*,*,#14143,.F.);
#18745=ORIENTED_EDGE('',*,*,#14225,.T.);
#25299=CONICAL_SURFACE('',#27288,15.65,0.785398163397448);
#25300=CONICAL_SURFACE('',#27295,1.325,0.785398163397448);
#25301=CONICAL_SURFACE('',#27308,15.65,0.785398163397448);
#25302=CONICAL_SURFACE('',#27315,2.825,0.785398163397448);
#25303=CONICAL_SURFACE('',#27317,15.65,0.785398163397448);
#25304=CONICAL_SURFACE('',#27322,2.08,0.785398163397448);
#25305=CONICAL_SURFACE('',#27334,15.65,0.785398163397448);
#25306=CONICAL_SURFACE('',#27336,2.075,0.785398163397447);
#25307=CONICAL_SURFACE('',#27349,3.575,0.785398163397447);
#25308=CONICAL_SURFACE('',#27354,15.5353553390593,1.17809724509618);
#25309=CONICAL_SURFACE('',#27357,15.5353553390593,1.17809724509617);
#25310=CONICAL_SURFACE('',#27360,15.5353553390593,1.17809724509617);
#25311=CONICAL_SURFACE('',#27362,15.5353553390593,1.17809724509616);
#25312=CONICAL_SURFACE('',#27365,2.8,0.785398163397448);
#25313=CONICAL_SURFACE('',#27368,3.55,0.785398163397451);
#25314=CONICAL_SURFACE('',#27371,1.3,0.785398163397448);
#25315=CONICAL_SURFACE('',#27374,2.05,0.785398163397451);
#25316=CONICAL_SURFACE('',#27377,15.65,0.785398163397448);
#25317=CONICAL_SURFACE('',#27378,15.65,0.785398163397448);
#25318=CONICAL_SURFACE('',#27381,2.055,0.785398163397448);
#25319=CONICAL_SURFACE('',#27384,15.65,0.785398163397448);
#25320=CONICAL_SURFACE('',#27388,15.65,0.785398163397448);
#25546=ADVANCED_FACE('',(#2733),#1727,.T.);
#25547=ADVANCED_FACE('',(#2734),#587,.T.);
#25548=ADVANCED_FACE('',(#2735),#25299,.T.);
#25549=ADVANCED_FACE('',(#2736),#1728,.T.);
#25550=ADVANCED_FACE('',(#2737),#1729,.T.);
#25551=ADVANCED_FACE('',(#2738),#1730,.T.);
#25552=ADVANCED_FACE('',(#2739),#1731,.F.);
#25553=ADVANCED_FACE('',(#2740),#1732,.T.);
#25554=ADVANCED_FACE('',(#2741),#25300,.F.);
#25555=ADVANCED_FACE('',(#2742),#1733,.T.);
#25556=ADVANCED_FACE('',(#2743,#850),#1734,.F.);
#25557=ADVANCED_FACE('',(#2744),#25301,.T.);
#25558=ADVANCED_FACE('',(#2745),#1735,.T.);
#25559=ADVANCED_FACE('',(#2746),#1736,.T.);
#25560=ADVANCED_FACE('',(#2747),#1737,.F.);
#25561=ADVANCED_FACE('',(#2748),#1738,.T.);
#25562=ADVANCED_FACE('',(#2749),#1739,.T.);
#25563=ADVANCED_FACE('',(#2750),#1740,.T.);
#25564=ADVANCED_FACE('',(#2751),#25302,.F.);
#25565=ADVANCED_FACE('',(#2752),#25303,.T.);
#25566=ADVANCED_FACE('',(#2753),#588,.F.);
#25567=ADVANCED_FACE('',(#2754),#1741,.F.);
#25568=ADVANCED_FACE('',(#2755),#25304,.F.);
#25569=ADVANCED_FACE('',(#2756),#589,.F.);
#25570=ADVANCED_FACE('',(#2757),#1742,.T.);
#25571=ADVANCED_FACE('',(#2758),#1743,.T.);
#25572=ADVANCED_FACE('',(#2759),#1744,.F.);
#25573=ADVANCED_FACE('',(#2760),#1745,.T.);
#25574=ADVANCED_FACE('',(#2761),#1746,.T.);
#25575=ADVANCED_FACE('',(#2762),#590,.T.);
#25576=ADVANCED_FACE('',(#2763),#25305,.T.);
#25577=ADVANCED_FACE('',(#2764),#1747,.T.);
#25578=ADVANCED_FACE('',(#2765),#25306,.F.);
#25579=ADVANCED_FACE('',(#2766),#591,.F.);
#25580=ADVANCED_FACE('',(#2767),#1748,.F.);
#25581=ADVANCED_FACE('',(#2768),#1749,.T.);
#25582=ADVANCED_FACE('',(#2769),#1750,.T.);
#25583=ADVANCED_FACE('',(#2770),#1751,.F.);
#25584=ADVANCED_FACE('',(#2771),#1752,.T.);
#25585=ADVANCED_FACE('',(#2772),#1753,.T.);
#25586=ADVANCED_FACE('',(#2773),#592,.T.);
#25587=ADVANCED_FACE('',(#2774),#1754,.T.);
#25588=ADVANCED_FACE('',(#2775),#25307,.F.);
#25589=ADVANCED_FACE('',(#2776),#593,.F.);
#25590=ADVANCED_FACE('',(#2777),#1755,.F.);
#25591=ADVANCED_FACE('',(#2778),#25308,.T.);
#25592=ADVANCED_FACE('',(#2779),#25309,.T.);
#25593=ADVANCED_FACE('',(#2780),#25310,.T.);
#25594=ADVANCED_FACE('',(#2781),#25311,.T.);
#25595=ADVANCED_FACE('',(#2782),#25312,.F.);
#25596=ADVANCED_FACE('',(#2783),#1756,.T.);
#25597=ADVANCED_FACE('',(#2784),#25313,.F.);
#25598=ADVANCED_FACE('',(#2785),#1757,.T.);
#25599=ADVANCED_FACE('',(#2786),#25314,.F.);
#25600=ADVANCED_FACE('',(#2787),#25315,.F.);
#25601=ADVANCED_FACE('',(#2788),#1758,.T.);
#25602=ADVANCED_FACE('',(#2789),#25316,.T.);
#25603=ADVANCED_FACE('',(#2790),#25317,.T.);
#25604=ADVANCED_FACE('',(#2791,#851),#1759,.T.);
#25605=ADVANCED_FACE('',(#2792),#25318,.F.);
#25606=ADVANCED_FACE('',(#2793),#594,.F.);
#25607=ADVANCED_FACE('',(#2794),#1760,.F.);
#25608=ADVANCED_FACE('',(#2795),#25319,.T.);
#25609=ADVANCED_FACE('',(#2796),#595,.T.);
#25610=ADVANCED_FACE('',(#2797),#25320,.T.);
#26874=CLOSED_SHELL('',(#25546,#25547,#25548,#25549,#25550,#25551,#25552,
#25553,#25554,#25555,#25556,#25557,#25558,#25559,#25560,#25561,#25562,#25563,
#25564,#25565,#25566,#25567,#25568,#25569,#25570,#25571,#25572,#25573,#25574,
#25575,#25576,#25577,#25578,#25579,#25580,#25581,#25582,#25583,#25584,#25585,
#25586,#25587,#25588,#25589,#25590,#25591,#25592,#25593,#25594,#25595,#25596,
#25597,#25598,#25599,#25600,#25601,#25602,#25603,#25604,#25605,#25606,#25607,
#25608,#25609,#25610));
#27283=AXIS2_PLACEMENT_3D('',#43621,#29629,#29630);
#27284=AXIS2_PLACEMENT_3D('',#43622,#29631,#29632);
#27285=AXIS2_PLACEMENT_3D('',#43639,#29637,#29638);
#27286=AXIS2_PLACEMENT_3D('',#43641,#29639,#29640);
#27287=AXIS2_PLACEMENT_3D('',#43644,#29642,#29643);
#27288=AXIS2_PLACEMENT_3D('',#43645,#29644,#29645);
#27289=AXIS2_PLACEMENT_3D('',#43651,#29646,#29647);
#27290=AXIS2_PLACEMENT_3D('',#43659,#29648,#29649);
#27291=AXIS2_PLACEMENT_3D('',#43670,#29653,#29654);
#27292=AXIS2_PLACEMENT_3D('',#43687,#29659,#29660);
#27293=AXIS2_PLACEMENT_3D('',#43697,#29664,#29665);
#27294=AXIS2_PLACEMENT_3D('',#43701,#29668,#29669);
#27295=AXIS2_PLACEMENT_3D('',#43714,#29672,#29673);
#27296=AXIS2_PLACEMENT_3D('',#43718,#29675,#29676);
#27297=AXIS2_PLACEMENT_3D('',#43719,#29677,#29678);
#27298=AXIS2_PLACEMENT_3D('',#43720,#29679,#29680);
#27299=AXIS2_PLACEMENT_3D('',#43727,#29683,#29684);
#27300=AXIS2_PLACEMENT_3D('',#43729,#29685,#29686);
#27301=AXIS2_PLACEMENT_3D('',#43733,#29688,#29689);
#27302=AXIS2_PLACEMENT_3D('',#43737,#29691,#29692);
#27303=AXIS2_PLACEMENT_3D('',#43741,#29694,#29695);
#27304=AXIS2_PLACEMENT_3D('',#43745,#29697,#29698);
#27305=AXIS2_PLACEMENT_3D('',#43749,#29700,#29701);
#27306=AXIS2_PLACEMENT_3D('',#43752,#29703,#29704);
#27307=AXIS2_PLACEMENT_3D('',#43754,#29705,#29706);
#27308=AXIS2_PLACEMENT_3D('',#43755,#29707,#29708);
#27309=AXIS2_PLACEMENT_3D('',#43763,#29709,#29710);
#27310=AXIS2_PLACEMENT_3D('',#43780,#29715,#29716);
#27311=AXIS2_PLACEMENT_3D('',#43795,#29720,#29721);
#27312=AXIS2_PLACEMENT_3D('',#43799,#29724,#29725);
#27313=AXIS2_PLACEMENT_3D('',#43804,#29727,#29728);
#27314=AXIS2_PLACEMENT_3D('',#43810,#29732,#29733);
#27315=AXIS2_PLACEMENT_3D('',#43814,#29736,#29737);
#27316=AXIS2_PLACEMENT_3D('',#43815,#29738,#29739);
#27317=AXIS2_PLACEMENT_3D('',#43816,#29740,#29741);
#27318=AXIS2_PLACEMENT_3D('',#43818,#29742,#29743);
#27319=AXIS2_PLACEMENT_3D('',#43826,#29744,#29745);
#27320=AXIS2_PLACEMENT_3D('',#43829,#29747,#29748);
#27321=AXIS2_PLACEMENT_3D('',#43830,#29749,#29750);
#27322=AXIS2_PLACEMENT_3D('',#43832,#29752,#29753);
#27323=AXIS2_PLACEMENT_3D('',#43835,#29755,#29756);
#27324=AXIS2_PLACEMENT_3D('',#43836,#29757,#29758);
#27325=AXIS2_PLACEMENT_3D('',#43838,#29759,#29760);
#27326=AXIS2_PLACEMENT_3D('',#43840,#29762,#29763);
#27327=AXIS2_PLACEMENT_3D('',#43857,#29768,#29769);
#27328=AXIS2_PLACEMENT_3D('',#43872,#29773,#29774);
#27329=AXIS2_PLACEMENT_3D('',#43876,#29777,#29778);
#27330=AXIS2_PLACEMENT_3D('',#43881,#29780,#29781);
#27331=AXIS2_PLACEMENT_3D('',#43898,#29786,#29787);
#27332=AXIS2_PLACEMENT_3D('',#43900,#29788,#29789);
#27333=AXIS2_PLACEMENT_3D('',#43903,#29791,#29792);
#27334=AXIS2_PLACEMENT_3D('',#43904,#29793,#29794);
#27335=AXIS2_PLACEMENT_3D('',#43915,#29795,#29796);
#27336=AXIS2_PLACEMENT_3D('',#43919,#29799,#29800);
#27337=AXIS2_PLACEMENT_3D('',#43920,#29801,#29802);
#27338=AXIS2_PLACEMENT_3D('',#43921,#29803,#29804);
#27339=AXIS2_PLACEMENT_3D('',#43924,#29806,#29807);
#27340=AXIS2_PLACEMENT_3D('',#43925,#29808,#29809);
#27341=AXIS2_PLACEMENT_3D('',#43927,#29811,#29812);
#27342=AXIS2_PLACEMENT_3D('',#43937,#29816,#29817);
#27343=AXIS2_PLACEMENT_3D('',#43952,#29821,#29822);
#27344=AXIS2_PLACEMENT_3D('',#43956,#29825,#29826);
#27345=AXIS2_PLACEMENT_3D('',#43958,#29828,#29829);
#27346=AXIS2_PLACEMENT_3D('',#43970,#29834,#29835);
#27347=AXIS2_PLACEMENT_3D('',#43971,#29836,#29837);
#27348=AXIS2_PLACEMENT_3D('',#43972,#29838,#29839);
#27349=AXIS2_PLACEMENT_3D('',#43976,#29842,#29843);
#27350=AXIS2_PLACEMENT_3D('',#43977,#29844,#29845);
#27351=AXIS2_PLACEMENT_3D('',#43978,#29846,#29847);
#27352=AXIS2_PLACEMENT_3D('',#43981,#29849,#29850);
#27353=AXIS2_PLACEMENT_3D('',#43982,#29851,#29852);
#27354=AXIS2_PLACEMENT_3D('',#43984,#29854,#29855);
#27355=AXIS2_PLACEMENT_3D('',#43985,#29856,#29857);
#27356=AXIS2_PLACEMENT_3D('',#43986,#29858,#29859);
#27357=AXIS2_PLACEMENT_3D('',#43987,#29860,#29861);
#27358=AXIS2_PLACEMENT_3D('',#43989,#29862,#29863);
#27359=AXIS2_PLACEMENT_3D('',#43991,#29864,#29865);
#27360=AXIS2_PLACEMENT_3D('',#43996,#29866,#29867);
#27361=AXIS2_PLACEMENT_3D('',#43998,#29868,#29869);
#27362=AXIS2_PLACEMENT_3D('',#44003,#29870,#29871);
#27363=AXIS2_PLACEMENT_3D('',#44005,#29872,#29873);
#27364=AXIS2_PLACEMENT_3D('',#44007,#29874,#29875);
#27365=AXIS2_PLACEMENT_3D('',#44012,#29876,#29877);
#27366=AXIS2_PLACEMENT_3D('',#44015,#29879,#29880);
#27367=AXIS2_PLACEMENT_3D('',#44016,#29881,#29882);
#27368=AXIS2_PLACEMENT_3D('',#44018,#29884,#29885);
#27369=AXIS2_PLACEMENT_3D('',#44021,#29887,#29888);
#27370=AXIS2_PLACEMENT_3D('',#44022,#29889,#29890);
#27371=AXIS2_PLACEMENT_3D('',#44027,#29892,#29893);
#27372=AXIS2_PLACEMENT_3D('',#44028,#29894,#29895);
#27373=AXIS2_PLACEMENT_3D('',#44029,#29896,#29897);
#27374=AXIS2_PLACEMENT_3D('',#44030,#29898,#29899);
#27375=AXIS2_PLACEMENT_3D('',#44033,#29901,#29902);
#27376=AXIS2_PLACEMENT_3D('',#44034,#29903,#29904);
#27377=AXIS2_PLACEMENT_3D('',#44039,#29906,#29907);
#27378=AXIS2_PLACEMENT_3D('',#44040,#29908,#29909);
#27379=AXIS2_PLACEMENT_3D('',#44041,#29910,#29911);
#27380=AXIS2_PLACEMENT_3D('',#44043,#29912,#29913);
#27381=AXIS2_PLACEMENT_3D('',#44044,#29914,#29915);
#27382=AXIS2_PLACEMENT_3D('',#44046,#29917,#29918);
#27383=AXIS2_PLACEMENT_3D('',#44048,#29920,#29921);
#27384=AXIS2_PLACEMENT_3D('',#44049,#29922,#29923);
#27385=AXIS2_PLACEMENT_3D('',#44050,#29924,#29925);
#27386=AXIS2_PLACEMENT_3D('',#44051,#29926,#29927);
#27387=AXIS2_PLACEMENT_3D('',#44052,#29928,#29929);
#27388=AXIS2_PLACEMENT_3D('',#44053,#29930,#29931);
#29629=DIRECTION('axis',(0.,0.,1.));
#29630=DIRECTION('refdir',(1.,0.,0.));
#29631=DIRECTION('center_axis',(-0.676715943576134,0.736244206571341,0.));
#29632=DIRECTION('ref_axis',(0.,0.,1.));
#29633=DIRECTION('',(0.,0.,-1.));
#29634=DIRECTION('',(-0.592886939594824,-0.54494967998502,0.592886939594817));
#29635=DIRECTION('',(0.,0.,1.));
#29636=DIRECTION('',(0.592886939594818,0.544949679985014,0.592886939594828));
#29637=DIRECTION('center_axis',(0.,0.,1.));
#29638=DIRECTION('ref_axis',(1.,0.,0.));
#29639=DIRECTION('center_axis',(0.,0.,1.));
#29640=DIRECTION('ref_axis',(1.,0.,0.));
#29641=DIRECTION('',(0.,0.,1.));
#29642=DIRECTION('center_axis',(0.,0.,-1.));
#29643=DIRECTION('ref_axis',(1.,0.,0.));
#29644=DIRECTION('center_axis',(0.,0.,-1.));
#29645=DIRECTION('ref_axis',(1.,0.,0.));
#29646=DIRECTION('center_axis',(0.,0.,1.));
#29647=DIRECTION('ref_axis',(1.,6.12323399573677E-17,0.));
#29648=DIRECTION('center_axis',(-0.707106781186554,1.3579178021049E-16,
0.707106781186541));
#29649=DIRECTION('ref_axis',(0.707106781186541,0.,0.707106781186554));
#29650=DIRECTION('',(-1.9203857723246E-16,-1.,0.));
#29651=DIRECTION('',(0.707106781186541,0.,0.707106781186554));
#29652=DIRECTION('',(1.9203857723246E-16,1.,0.));
#29653=DIRECTION('center_axis',(0.676715943576129,0.736244206571345,0.));
#29654=DIRECTION('ref_axis',(0.,0.,-1.));
#29655=DIRECTION('',(0.,0.,1.));
#29656=DIRECTION('',(0.59288693959482,-0.54494967998501,-0.59288693959483));
#29657=DIRECTION('',(0.,0.,-1.));
#29658=DIRECTION('',(-0.592886939594826,0.544949679985016,-0.592886939594819));
#29659=DIRECTION('center_axis',(0.707106781186543,-1.35791780210488E-16,
-0.707106781186552));
#29660=DIRECTION('ref_axis',(-0.707106781186552,0.,-0.707106781186543));
#29661=DIRECTION('',(-1.9203857723246E-16,-1.,0.));
#29662=DIRECTION('',(-0.707106781186552,0.,-0.707106781186543));
#29663=DIRECTION('',(1.9203857723246E-16,1.,0.));
#29664=DIRECTION('center_axis',(-1.,1.9203857723246E-16,0.));
#29665=DIRECTION('ref_axis',(1.9203857723246E-16,1.,0.));
#29666=DIRECTION('',(1.9203857723246E-16,1.,0.));
#29667=DIRECTION('',(0.,0.,-1.));
#29668=DIRECTION('center_axis',(0.707106781186554,-1.3579178021049E-16,
0.707106781186541));
#29669=DIRECTION('ref_axis',(0.707106781186541,0.,-0.707106781186554));
#29670=DIRECTION('',(-1.9203857723246E-16,-1.,0.));
#29671=DIRECTION('',(-0.707106781186548,0.,0.707106781186548));
#29672=DIRECTION('center_axis',(0.,0.,-1.));
#29673=DIRECTION('ref_axis',(-1.,0.,0.));
#29674=DIRECTION('',(0.707106781186548,0.,-0.707106781186548));
#29675=DIRECTION('center_axis',(0.,0.,-1.));
#29676=DIRECTION('ref_axis',(-1.,0.,0.));
#29677=DIRECTION('center_axis',(0.,0.,1.));
#29678=DIRECTION('ref_axis',(-1.,0.,0.));
#29679=DIRECTION('center_axis',(-0.707106781186543,1.35791780210488E-16,
-0.707106781186552));
#29680=DIRECTION('ref_axis',(-0.707106781186552,0.,0.707106781186543));
#29681=DIRECTION('',(-1.9203857723246E-16,-1.,0.));
#29682=DIRECTION('',(1.9203857723246E-16,1.,0.));
#29683=DIRECTION('center_axis',(0.,0.,1.));
#29684=DIRECTION('ref_axis',(1.,0.,0.));
#29685=DIRECTION('center_axis',(0.,0.,1.));
#29686=DIRECTION('ref_axis',(1.,0.,0.));
#29687=DIRECTION('',(1.,0.,0.));
#29688=DIRECTION('center_axis',(0.,0.,-1.));
#29689=DIRECTION('ref_axis',(0.,1.,0.));
#29690=DIRECTION('',(-1.,0.,0.));
#29691=DIRECTION('center_axis',(0.,0.,1.));
#29692=DIRECTION('ref_axis',(1.,0.,0.));
#29693=DIRECTION('',(-1.9203857723246E-16,-1.,0.));
#29694=DIRECTION('center_axis',(0.,0.,-1.));
#29695=DIRECTION('ref_axis',(1.,0.,0.));
#29696=DIRECTION('',(1.44028932924345E-16,1.,0.));
#29697=DIRECTION('center_axis',(0.,0.,1.));
#29698=DIRECTION('ref_axis',(1.,0.,0.));
#29699=DIRECTION('',(-1.,1.20024110770287E-16,0.));
#29700=DIRECTION('center_axis',(0.,0.,-1.));
#29701=DIRECTION('ref_axis',(-2.88998133608509E-16,-1.,0.));
#29702=DIRECTION('',(1.,-1.44028932924345E-16,0.));
#29703=DIRECTION('center_axis',(0.,0.,1.));
#29704=DIRECTION('ref_axis',(1.,0.,0.));
#29705=DIRECTION('center_axis',(0.,0.,-1.));
#29706=DIRECTION('ref_axis',(1.,0.,0.));
#29707=DIRECTION('center_axis',(0.,0.,1.));
#29708=DIRECTION('ref_axis',(1.,0.,0.));
#29709=DIRECTION('center_axis',(0.76788343892593,0.640589591098144,0.));
#29710=DIRECTION('ref_axis',(0.,0.,-1.));
#29711=DIRECTION('',(0.,0.,-1.));
#29712=DIRECTION('',(-0.508077317375032,0.609039177544843,0.609039177544837));
#29713=DIRECTION('',(0.,0.,1.));
#29714=DIRECTION('',(0.508077317375028,-0.609039177544838,0.609039177544846));
#29715=DIRECTION('center_axis',(0.,0.707106781186552,0.707106781186543));
#29716=DIRECTION('ref_axis',(1.,0.,0.));
#29717=DIRECTION('',(-1.,0.,0.));
#29718=DIRECTION('',(0.,-0.707106781186543,0.707106781186552));
#29719=DIRECTION('',(1.,0.,0.));
#29720=DIRECTION('center_axis',(0.,-1.,0.));
#29721=DIRECTION('ref_axis',(-1.,0.,0.));
#29722=DIRECTION('',(1.,0.,0.));
#29723=DIRECTION('',(0.,0.,-1.));
#29724=DIRECTION('center_axis',(0.,0.707106781186544,-0.707106781186551));
#29725=DIRECTION('ref_axis',(-1.,0.,0.));
#29726=DIRECTION('',(0.,-0.707106781186548,-0.707106781186548));
#29727=DIRECTION('center_axis',(0.76788343892593,-0.640589591098144,0.));
#29728=DIRECTION('ref_axis',(0.,0.,-1.));
#29729=DIRECTION('',(-0.508077317375028,-0.609039177544838,-0.609039177544846));
#29730=DIRECTION('',(0.,0.,-1.));
#29731=DIRECTION('',(0.508077317375032,0.609039177544843,-0.609039177544837));
#29732=DIRECTION('center_axis',(0.,-0.707106781186544,-0.707106781186551));
#29733=DIRECTION('ref_axis',(-1.,0.,0.));
#29734=DIRECTION('',(-1.,0.,0.));
#29735=DIRECTION('',(0.,0.707106781186551,-0.707106781186544));
#29736=DIRECTION('center_axis',(0.,0.,-1.));
#29737=DIRECTION('ref_axis',(0.,1.,0.));
#29738=DIRECTION('center_axis',(0.,0.,1.));
#29739=DIRECTION('ref_axis',(0.,1.,0.));
#29740=DIRECTION('center_axis',(0.,0.,1.));
#29741=DIRECTION('ref_axis',(1.,0.,0.));
#29742=DIRECTION('center_axis',(0.,0.,-1.));
#29743=DIRECTION('ref_axis',(1.,0.,0.));
#29744=DIRECTION('center_axis',(0.,0.,-1.));
#29745=DIRECTION('ref_axis',(0.,1.,0.));
#29746=DIRECTION('',(0.,0.,-1.));
#29747=DIRECTION('center_axis',(0.,0.,-1.));
#29748=DIRECTION('ref_axis',(0.,1.,0.));
#29749=DIRECTION('center_axis',(0.,1.,0.));
#29750=DIRECTION('ref_axis',(1.,0.,0.));
#29751=DIRECTION('',(1.,0.,0.));
#29752=DIRECTION('center_axis',(0.,0.,-1.));
#29753=DIRECTION('ref_axis',(1.,0.,0.));
#29754=DIRECTION('',(0.707106781186548,-8.65956056235493E-17,0.707106781186548));
#29755=DIRECTION('center_axis',(0.,0.,1.));
#29756=DIRECTION('ref_axis',(1.,0.,0.));
#29757=DIRECTION('center_axis',(0.,0.,-1.));
#29758=DIRECTION('ref_axis',(1.,0.,0.));
#29759=DIRECTION('center_axis',(0.,0.,-1.));
#29760=DIRECTION('ref_axis',(1.,0.,0.));
#29761=DIRECTION('',(0.,0.,-1.));
#29762=DIRECTION('center_axis',(-0.752232026437047,-0.658898306571215,0.));
#29763=DIRECTION('ref_axis',(0.,0.,1.));
#29764=DIRECTION('',(0.,0.,-1.));
#29765=DIRECTION('',(0.526553973041879,-0.601140962451329,0.601140962451322));
#29766=DIRECTION('',(0.,0.,1.));
#29767=DIRECTION('',(-0.526553973041875,0.601140962451325,0.60114096245133));
#29768=DIRECTION('center_axis',(-1.01843835157867E-16,-0.707106781186551,
0.707106781186544));
#29769=DIRECTION('ref_axis',(1.,0.,1.44028932924346E-16));
#29770=DIRECTION('',(1.,-1.44028932924345E-16,0.));
#29771=DIRECTION('',(-3.23639307574421E-16,0.707106781186544,0.707106781186551));
#29772=DIRECTION('',(-1.,1.44028932924345E-16,0.));
#29773=DIRECTION('center_axis',(1.44028932924345E-16,1.,0.));
#29774=DIRECTION('ref_axis',(1.,-1.44028932924345E-16,0.));
#29775=DIRECTION('',(-1.,1.44028932924345E-16,0.));
#29776=DIRECTION('',(0.,0.,-1.));
#29777=DIRECTION('center_axis',(-1.01843835157866E-16,-0.707106781186543,
-0.707106781186552));
#29778=DIRECTION('ref_axis',(-1.,0.,1.44028932924343E-16));
#29779=DIRECTION('',(2.9094814564838E-16,0.707106781186548,-0.707106781186548));
#29780=DIRECTION('center_axis',(-0.752232026437047,0.658898306571214,0.));
#29781=DIRECTION('ref_axis',(0.,0.,1.));
#29782=DIRECTION('',(0.,0.,1.));
#29783=DIRECTION('',(0.526553973041873,0.601140962451323,-0.601140962451333));
#29784=DIRECTION('',(0.,0.,-1.));
#29785=DIRECTION('',(-0.526553973041878,-0.601140962451329,-0.601140962451323));
#29786=DIRECTION('center_axis',(0.,0.,1.));
#29787=DIRECTION('ref_axis',(1.,0.,0.));
#29788=DIRECTION('center_axis',(0.,0.,-1.));
#29789=DIRECTION('ref_axis',(1.,0.,0.));
#29790=DIRECTION('',(0.,0.,-1.));
#29791=DIRECTION('center_axis',(0.,0.,1.));
#29792=DIRECTION('ref_axis',(1.,0.,0.));
#29793=DIRECTION('center_axis',(0.,0.,1.));
#29794=DIRECTION('ref_axis',(1.,0.,0.));
#29795=DIRECTION('center_axis',(8.4869862631555E-17,0.707106781186544,-0.707106781186551));
#29796=DIRECTION('ref_axis',(-1.,0.,-1.20024110770286E-16));
#29797=DIRECTION('',(1.,-1.20024110770287E-16,0.));
#29798=DIRECTION('',(-9.38848536597713E-16,-0.707106781186551,-0.707106781186544));
#29799=DIRECTION('center_axis',(0.,0.,-1.));
#29800=DIRECTION('ref_axis',(-2.88998133608509E-16,-1.,0.));
#29801=DIRECTION('center_axis',(0.,0.,1.));
#29802=DIRECTION('ref_axis',(-2.88998133608509E-16,-1.,0.));
#29803=DIRECTION('center_axis',(0.,0.,-1.));
#29804=DIRECTION('ref_axis',(-2.88998133608509E-16,-1.,0.));
#29805=DIRECTION('',(0.,0.,-1.));
#29806=DIRECTION('center_axis',(0.,0.,-1.));
#29807=DIRECTION('ref_axis',(-2.88998133608509E-16,-1.,0.));
#29808=DIRECTION('center_axis',(-1.20024110770287E-16,-1.,0.));
#29809=DIRECTION('ref_axis',(-1.,1.20024110770287E-16,0.));
#29810=DIRECTION('',(-1.,1.20024110770287E-16,0.));
#29811=DIRECTION('center_axis',(0.621746515478052,-0.783218533035895,0.));
#29812=DIRECTION('ref_axis',(0.,0.,-1.));
#29813=DIRECTION('',(0.616605963274096,0.48948357695602,0.616605963274087));
#29814=DIRECTION('',(0.,0.,1.));
#29815=DIRECTION('',(-0.616605963274091,-0.489483576956017,0.616605963274094));
#29816=DIRECTION('center_axis',(0.707106781186549,-1.01843835157867E-16,
0.707106781186546));
#29817=DIRECTION('ref_axis',(0.707106781186546,0.,-0.707106781186549));
#29818=DIRECTION('',(1.44028932924345E-16,1.,0.));
#29819=DIRECTION('',(-0.707106781186544,0.,0.707106781186551));
#29820=DIRECTION('',(-1.44028932924345E-16,-1.,0.));
#29821=DIRECTION('center_axis',(-1.,1.44028932924345E-16,0.));
#29822=DIRECTION('ref_axis',(1.44028932924345E-16,1.,0.));
#29823=DIRECTION('',(-1.44028932924345E-16,-1.,0.));
#29824=DIRECTION('',(0.,0.,-1.));
#29825=DIRECTION('center_axis',(0.707106781186542,-1.01843835157866E-16,
-0.707106781186553));
#29826=DIRECTION('ref_axis',(-0.707106781186553,0.,-0.707106781186542));
#29827=DIRECTION('',(-0.707106781186546,4.18691322315673E-15,-0.707106781186549));
#29828=DIRECTION('center_axis',(-0.621746515478056,-0.783218533035893,0.));
#29829=DIRECTION('ref_axis',(0.,0.,1.));
#29830=DIRECTION('',(0.,0.,1.));
#29831=DIRECTION('',(-0.616605963274087,0.489483576956018,-0.616605963274098));
#29832=DIRECTION('',(0.,0.,-1.));
#29833=DIRECTION('',(0.616605963274094,-0.489483576956023,-0.616605963274087));
#29834=DIRECTION('center_axis',(0.,0.,1.));
#29835=DIRECTION('ref_axis',(1.,0.,0.));
#29836=DIRECTION('center_axis',(0.,0.,1.));
#29837=DIRECTION('ref_axis',(1.,0.,0.));
#29838=DIRECTION('center_axis',(-0.707106781186543,1.35791780210488E-16,
-0.707106781186552));
#29839=DIRECTION('ref_axis',(-0.707106781186552,0.,0.707106781186543));
#29840=DIRECTION('',(1.9203857723246E-16,1.,0.));
#29841=DIRECTION('',(0.707106781186552,0.,-0.707106781186543));
#29842=DIRECTION('center_axis',(0.,0.,-1.));
#29843=DIRECTION('ref_axis',(1.,0.,0.));
#29844=DIRECTION('center_axis',(0.,0.,1.));
#29845=DIRECTION('ref_axis',(1.,0.,0.));
#29846=DIRECTION('center_axis',(0.,0.,-1.));
#29847=DIRECTION('ref_axis',(1.,0.,0.));
#29848=DIRECTION('',(0.,0.,-1.));
#29849=DIRECTION('center_axis',(0.,0.,-1.));
#29850=DIRECTION('ref_axis',(1.,0.,0.));
#29851=DIRECTION('center_axis',(1.,-1.9203857723246E-16,0.));
#29852=DIRECTION('ref_axis',(-1.9203857723246E-16,-1.,0.));
#29853=DIRECTION('',(-1.9203857723246E-16,-1.,0.));
#29854=DIRECTION('center_axis',(0.,-1.35268490144193E-14,-1.));
#29855=DIRECTION('ref_axis',(-1.,-3.07843832903329E-17,0.));
#29856=DIRECTION('center_axis',(0.,0.,-1.));
#29857=DIRECTION('ref_axis',(-1.,0.,0.));
#29858=DIRECTION('center_axis',(0.,0.,1.));
#29859=DIRECTION('ref_axis',(-1.,-6.12323399573677E-17,0.));
#29860=DIRECTION('center_axis',(0.,-1.35268490144193E-14,-1.));
#29861=DIRECTION('ref_axis',(-1.,-3.07843832903329E-17,0.));
#29862=DIRECTION('center_axis',(0.,0.,1.));
#29863=DIRECTION('ref_axis',(-1.,-6.12323399573677E-17,0.));
#29864=DIRECTION('center_axis',(0.,0.,-1.));
#29865=DIRECTION('ref_axis',(-1.,0.,0.));
#29866=DIRECTION('center_axis',(-2.51214793389404E-14,-1.35268490144193E-14,
-1.));
#29867=DIRECTION('ref_axis',(1.,3.07843832903329E-17,0.));
#29868=DIRECTION('center_axis',(0.,0.,-1.));
#29869=DIRECTION('ref_axis',(1.,0.,0.));
#29870=DIRECTION('center_axis',(1.25607396694696E-14,-1.35268490144186E-14,
-1.));
#29871=DIRECTION('ref_axis',(1.,3.07843832903329E-17,0.));
#29872=DIRECTION('center_axis',(-6.96322261624857E-33,1.13718055215539E-16,
1.));
#29873=DIRECTION('ref_axis',(1.,6.12323399573677E-17,0.));
#29874=DIRECTION('center_axis',(0.,0.,-1.));
#29875=DIRECTION('ref_axis',(1.,0.,0.));
#29876=DIRECTION('center_axis',(0.,0.,1.));
#29877=DIRECTION('ref_axis',(0.,1.,0.));
#29878=DIRECTION('',(0.,0.707106781186548,0.707106781186548));
#29879=DIRECTION('center_axis',(0.,0.,1.));
#29880=DIRECTION('ref_axis',(0.,1.,0.));
#29881=DIRECTION('center_axis',(0.,-0.707106781186552,0.707106781186543));
#29882=DIRECTION('ref_axis',(1.,0.,0.));
#29883=DIRECTION('',(-1.,0.,0.));
#29884=DIRECTION('center_axis',(0.,0.,1.));
#29885=DIRECTION('ref_axis',(1.,0.,0.));
#29886=DIRECTION('',(0.707106781186548,6.28036983473512E-15,0.707106781186548));
#29887=DIRECTION('center_axis',(0.,0.,1.));
#29888=DIRECTION('ref_axis',(1.,0.,0.));
#29889=DIRECTION('center_axis',(-0.707106781186554,1.3579178021049E-16,
0.707106781186541));
#29890=DIRECTION('ref_axis',(0.707106781186541,0.,0.707106781186554));
#29891=DIRECTION('',(1.9203857723246E-16,1.,0.));
#29892=DIRECTION('center_axis',(0.,0.,1.));
#29893=DIRECTION('ref_axis',(-1.,0.,0.));
#29894=DIRECTION('center_axis',(0.,0.,1.));
#29895=DIRECTION('ref_axis',(-1.,0.,0.));
#29896=DIRECTION('center_axis',(0.,0.,-1.));
#29897=DIRECTION('ref_axis',(-1.,0.,0.));
#29898=DIRECTION('center_axis',(0.,0.,1.));
#29899=DIRECTION('ref_axis',(-2.88998133608509E-16,-1.,0.));
#29900=DIRECTION('',(3.43266289616425E-15,-0.707106781186548,0.707106781186547));
#29901=DIRECTION('center_axis',(0.,0.,1.));
#29902=DIRECTION('ref_axis',(-2.88998133608509E-16,-1.,0.));
#29903=DIRECTION('center_axis',(8.48698626315561E-17,0.707106781186553,
0.707106781186542));
#29904=DIRECTION('ref_axis',(1.,0.,-1.20024110770289E-16));
#29905=DIRECTION('',(1.,-1.20024110770287E-16,0.));
#29906=DIRECTION('center_axis',(0.,0.,-1.));
#29907=DIRECTION('ref_axis',(1.,0.,0.));
#29908=DIRECTION('center_axis',(0.,0.,-1.));
#29909=DIRECTION('ref_axis',(1.,0.,0.));
#29910=DIRECTION('center_axis',(0.,0.,1.));
#29911=DIRECTION('ref_axis',(1.,0.,0.));
#29912=DIRECTION('center_axis',(0.,0.,1.));
#29913=DIRECTION('ref_axis',(1.,0.,0.));
#29914=DIRECTION('center_axis',(0.,0.,1.));
#29915=DIRECTION('ref_axis',(1.,0.,0.));
#29916=DIRECTION('',(0.707106781186548,8.65956056235493E-17,-0.707106781186548));
#29917=DIRECTION('center_axis',(0.,0.,-1.));
#29918=DIRECTION('ref_axis',(-1.,0.,0.));
#29919=DIRECTION('',(0.,0.,-1.));
#29920=DIRECTION('center_axis',(1.,-1.9203857723246E-16,0.));
#29921=DIRECTION('ref_axis',(-1.9203857723246E-16,-1.,0.));
#29922=DIRECTION('center_axis',(0.,0.,-1.));
#29923=DIRECTION('ref_axis',(1.,0.,0.));
#29924=DIRECTION('center_axis',(0.,0.,1.));
#29925=DIRECTION('ref_axis',(1.,0.,0.));
#29926=DIRECTION('center_axis',(0.,0.,1.));
#29927=DIRECTION('ref_axis',(1.,0.,0.));
#29928=DIRECTION('center_axis',(0.,0.,-1.));
#29929=DIRECTION('ref_axis',(1.,0.,0.));
#29930=DIRECTION('center_axis',(0.,0.,1.));
#29931=DIRECTION('ref_axis',(1.,0.,0.));
#43621=CARTESIAN_POINT('',(0.,0.,0.));
#43622=CARTESIAN_POINT('Origin',(8.82473422894286,15.6190101383511,11.));
#43623=CARTESIAN_POINT('',(8.77479843761413,15.5731118537254,15.4247984376141));
#43624=CARTESIAN_POINT('',(8.89946845788571,15.6877018085946,15.3));
#43625=CARTESIAN_POINT('Ctrl Pts',(8.77479843761413,15.5731118537254,15.4247984376141));
#43626=CARTESIAN_POINT('Ctrl Pts',(8.8368855031481,15.6301789338622,15.3628561636274));
#43627=CARTESIAN_POINT('Ctrl Pts',(8.89946845788572,15.6877018085946,15.3));
#43628=CARTESIAN_POINT('',(8.89946845788571,15.6877018085946,11.2));
#43629=CARTESIAN_POINT('',(8.89946845788571,15.6877018085946,11.));
#43630=CARTESIAN_POINT('',(8.79981911738071,15.5961095123365,11.1001808826193));
#43631=CARTESIAN_POINT('Ctrl Pts',(8.89946845788572,15.6877018085946,11.2));
#43632=CARTESIAN_POINT('Ctrl Pts',(8.84948539827205,15.6417600775122,11.1497987369429));
#43633=CARTESIAN_POINT('Ctrl Pts',(8.79981911738071,15.5961095123365,11.1001808826193));
#43634=CARTESIAN_POINT('',(8.75,15.5503184681076,11.15));
#43635=CARTESIAN_POINT('',(7.66780970362768,14.5556275476194,12.2321902963723));
#43636=CARTESIAN_POINT('',(8.75,15.5503184681076,15.4));
#43637=CARTESIAN_POINT('',(8.75,15.5503184681076,11.));
#43638=CARTESIAN_POINT('',(6.85932538040084,13.8125123872206,13.5093253804008));
#43639=CARTESIAN_POINT('Origin',(7.5,0.,11.));
#43640=CARTESIAN_POINT('',(22.9811689265378,2.89756944144577,15.3));
#43641=CARTESIAN_POINT('Origin',(7.5,0.,15.3));
#43642=CARTESIAN_POINT('',(22.9811689265378,2.89756944144577,11.2));
#43643=CARTESIAN_POINT('',(22.9811689265378,2.89756944144577,11.));
#43644=CARTESIAN_POINT('Origin',(7.5,0.,11.2));
#43645=CARTESIAN_POINT('Origin',(7.5,0.,15.4));
#43646=CARTESIAN_POINT('',(8.77928932188135,15.5682375662889,15.4292893218813));
#43647=CARTESIAN_POINT('Ctrl Pts',(8.77928932188135,15.5682375662889,15.4292893218813));
#43648=CARTESIAN_POINT('Ctrl Pts',(8.77704423120747,15.5706747100072,15.4270442312075));
#43649=CARTESIAN_POINT('Ctrl Pts',(8.77479843761413,15.5731118537254,15.4247984376141));
#43650=CARTESIAN_POINT('',(22.8714720490513,2.77928932188135,15.4292893218813));
#43651=CARTESIAN_POINT('Origin',(7.5,-9.56492666618245E-16,15.4292893218813));
#43652=CARTESIAN_POINT('',(22.877968161414,2.77386128332979,15.4238612833298));
#43653=CARTESIAN_POINT('Ctrl Pts',(22.877968161414,2.77386128332979,15.4238612833298));
#43654=CARTESIAN_POINT('Ctrl Pts',(22.8747201052327,2.77657587596802,15.426575875968));
#43655=CARTESIAN_POINT('Ctrl Pts',(22.8714720490513,2.77928932188135,15.4292893218813));
#43656=CARTESIAN_POINT('Ctrl Pts',(22.9811689265378,2.89756944144577,15.3));
#43657=CARTESIAN_POINT('Ctrl Pts',(22.9293648449271,2.83547118557273,15.3623442379101));
#43658=CARTESIAN_POINT('Ctrl Pts',(22.877968161414,2.77386128332979,15.4238612833298));
#43659=CARTESIAN_POINT('Origin',(8.8,8.375,15.45));
#43660=CARTESIAN_POINT('',(8.75,7.5,15.4));
#43661=CARTESIAN_POINT('',(8.75,8.375,15.4));
#43662=CARTESIAN_POINT('',(8.85,7.5,15.5));
#43663=CARTESIAN_POINT('',(8.75,7.5,15.4));
#43664=CARTESIAN_POINT('',(8.85,15.3909064060568,15.5));
#43665=CARTESIAN_POINT('',(8.85,8.375,15.5));
#43666=CARTESIAN_POINT('Ctrl Pts',(8.77928932188134,15.5682375662889,15.4292893218812));
#43667=CARTESIAN_POINT('Ctrl Pts',(8.80288271557749,15.5091473511845,15.4528827155773));
#43668=CARTESIAN_POINT('Ctrl Pts',(8.826454184001,15.4500345909188,15.4764541840008));
#43669=CARTESIAN_POINT('Ctrl Pts',(8.84999999999999,15.3909064060567,15.4999999999998));
#43670=CARTESIAN_POINT('Origin',(6.17526577105714,15.6190101383511,11.));
#43671=CARTESIAN_POINT('',(6.20018088261929,15.5961095123365,11.1001808826193));
#43672=CARTESIAN_POINT('',(6.10053154211429,15.6877018085946,11.2));
#43673=CARTESIAN_POINT('Ctrl Pts',(6.20018088261929,15.5961095123365,11.1001808826193));
#43674=CARTESIAN_POINT('Ctrl Pts',(6.15051460172865,15.6417600775116,11.1497987369422));
#43675=CARTESIAN_POINT('Ctrl Pts',(6.10053154211428,15.6877018085946,11.2));
#43676=CARTESIAN_POINT('',(6.10053154211429,15.6877018085946,15.3));
#43677=CARTESIAN_POINT('',(6.10053154211429,15.6877018085946,11.));
#43678=CARTESIAN_POINT('',(6.22520156238587,15.5731118537254,15.4247984376141));
#43679=CARTESIAN_POINT('Ctrl Pts',(6.10053154211428,15.6877018085946,15.3));
#43680=CARTESIAN_POINT('Ctrl Pts',(6.16311449685252,15.6301789338617,15.362856163628));
#43681=CARTESIAN_POINT('Ctrl Pts',(6.22520156238587,15.5731118537254,15.4247984376141));
#43682=CARTESIAN_POINT('',(6.25,15.5503184681076,15.4));
#43683=CARTESIAN_POINT('',(8.88782844934798,13.1257689067529,12.762171550652));
#43684=CARTESIAN_POINT('',(6.25,15.5503184681076,11.15));
#43685=CARTESIAN_POINT('',(6.25,15.5503184681076,11.));
#43686=CARTESIAN_POINT('',(8.07934412612115,13.8688840671517,12.9793441261211));
#43687=CARTESIAN_POINT('Origin',(6.175,3.75,11.075));
#43688=CARTESIAN_POINT('',(6.25,7.5,11.15));
#43689=CARTESIAN_POINT('',(6.25,3.75,11.15));
#43690=CARTESIAN_POINT('',(6.1,7.5,11.));
#43691=CARTESIAN_POINT('',(6.25,7.5,11.15));
#43692=CARTESIAN_POINT('',(6.1,15.4868492599366,11.));
#43693=CARTESIAN_POINT('',(6.1,3.75,11.));
#43694=CARTESIAN_POINT('Ctrl Pts',(6.1,15.4868492599366,11.));
#43695=CARTESIAN_POINT('Ctrl Pts',(6.14991436752269,15.5414793861366,11.0499143675227));
#43696=CARTESIAN_POINT('Ctrl Pts',(6.20018088261929,15.5961095123365,11.1001808826193));
#43697=CARTESIAN_POINT('Origin',(6.25,7.5,15.5));
#43698=CARTESIAN_POINT('',(6.25,7.5,15.4));
#43699=CARTESIAN_POINT('',(6.25,3.75,15.4));
#43700=CARTESIAN_POINT('',(6.25,7.5,15.5));
#43701=CARTESIAN_POINT('Origin',(6.2,3.75,15.45));
#43702=CARTESIAN_POINT('',(6.22071067811865,15.568237566289,15.4292893218813));
#43703=CARTESIAN_POINT('Ctrl Pts',(6.22520156238587,15.5731118537254,15.4247984376141));
#43704=CARTESIAN_POINT('Ctrl Pts',(6.22295576879253,15.5706747100072,15.4270442312075));
#43705=CARTESIAN_POINT('Ctrl Pts',(6.22071067811865,15.568237566289,15.4292893218813));
#43706=CARTESIAN_POINT('',(6.15,15.3909064060568,15.5));
#43707=CARTESIAN_POINT('Ctrl Pts',(6.15000000000001,15.3909064060567,15.4999999999998));
#43708=CARTESIAN_POINT('Ctrl Pts',(6.17354581599823,15.4500345909168,15.4764541840016));
#43709=CARTESIAN_POINT('Ctrl Pts',(6.19711728442092,15.5091473511805,15.4528827155789));
#43710=CARTESIAN_POINT('Ctrl Pts',(6.22071067811866,15.5682375662889,15.4292893218812));
#43711=CARTESIAN_POINT('',(6.15,7.5,15.5));
#43712=CARTESIAN_POINT('',(6.15,3.75,15.5));
#43713=CARTESIAN_POINT('',(6.25,7.5,15.4));
#43714=CARTESIAN_POINT('Origin',(7.5,7.5,11.075));
#43715=CARTESIAN_POINT('',(8.75,7.5,11.15));
#43716=CARTESIAN_POINT('',(8.9,7.5,11.));
#43717=CARTESIAN_POINT('',(8.75,7.5,11.15));
#43718=CARTESIAN_POINT('Origin',(7.5,7.5,11.));
#43719=CARTESIAN_POINT('Origin',(7.5,7.5,11.15));
#43720=CARTESIAN_POINT('Origin',(8.825,8.375,11.075));
#43721=CARTESIAN_POINT('',(8.9,15.4868492599366,11.));
#43722=CARTESIAN_POINT('Ctrl Pts',(8.79981911738071,15.5961095123365,11.1001808826193));
#43723=CARTESIAN_POINT('Ctrl Pts',(8.85008563247733,15.5414793861366,11.0499143675227));
#43724=CARTESIAN_POINT('Ctrl Pts',(8.9,15.4868492599366,11.));
#43725=CARTESIAN_POINT('',(8.9,8.375,11.));
#43726=CARTESIAN_POINT('',(8.75,8.375,11.15));
#43727=CARTESIAN_POINT('Origin',(7.5,0.,11.));
#43728=CARTESIAN_POINT('',(22.777188877539,2.9,11.));
#43729=CARTESIAN_POINT('Origin',(7.5,0.,11.));
#43730=CARTESIAN_POINT('',(15.,2.9,11.));
#43731=CARTESIAN_POINT('',(11.25,2.9,11.));
#43732=CARTESIAN_POINT('',(15.,-2.9,11.));
#43733=CARTESIAN_POINT('Origin',(15.,0.,11.));
#43734=CARTESIAN_POINT('',(22.777188877539,-2.9,11.));
#43735=CARTESIAN_POINT('',(15.875,-2.9,11.));
#43736=CARTESIAN_POINT('',(11.15,-15.1155549021529,11.));
#43737=CARTESIAN_POINT('Origin',(7.5,0.,11.));
#43738=CARTESIAN_POINT('',(11.15,-7.5,11.));
#43739=CARTESIAN_POINT('',(11.15,-3.75,11.));
#43740=CARTESIAN_POINT('',(3.85,-7.5,11.));
#43741=CARTESIAN_POINT('Origin',(7.5,-7.5,11.));
#43742=CARTESIAN_POINT('',(3.85,-15.1155549021529,11.));
#43743=CARTESIAN_POINT('',(3.85,-8.375,11.));
#43744=CARTESIAN_POINT('',(-7.90064933695979,-2.15,11.));
#43745=CARTESIAN_POINT('Origin',(7.5,0.,11.));
#43746=CARTESIAN_POINT('',(-4.44089209850063E-16,-2.15,11.));
#43747=CARTESIAN_POINT('',(3.75,-2.15,11.));
#43748=CARTESIAN_POINT('',(1.21771195646252E-15,2.15,11.));
#43749=CARTESIAN_POINT('Origin',(3.33066907387547E-16,1.11022302462516E-15,
11.));
#43750=CARTESIAN_POINT('',(-7.90064933695979,2.15,11.));
#43751=CARTESIAN_POINT('',(-0.875,2.15,11.));
#43752=CARTESIAN_POINT('Origin',(7.5,0.,11.));
#43753=CARTESIAN_POINT('',(5.345,2.63911385216255E-16,11.));
#43754=CARTESIAN_POINT('Origin',(7.5,0.,11.));
#43755=CARTESIAN_POINT('Origin',(7.5,0.,11.1));
#43756=CARTESIAN_POINT('',(22.8988337499022,2.79887314750332,11.1011268524967));
#43757=CARTESIAN_POINT('Ctrl Pts',(22.8988337499022,2.79887314750332,11.1011268524967));
#43758=CARTESIAN_POINT('Ctrl Pts',(22.9398717132847,2.84806591130492,11.1503003777304));
#43759=CARTESIAN_POINT('Ctrl Pts',(22.9811689265378,2.89756944144577,11.2));
#43760=CARTESIAN_POINT('Ctrl Pts',(22.777188877539,2.9,11.));
#43761=CARTESIAN_POINT('Ctrl Pts',(22.8380113137205,2.84963708154271,11.0503629184573));
#43762=CARTESIAN_POINT('Ctrl Pts',(22.8988337499022,2.79887314750332,11.1011268524967));
#43763=CARTESIAN_POINT('Origin',(22.9196156729043,-2.82378472072289,11.));
#43764=CARTESIAN_POINT('',(22.877968161414,-2.77386128332979,15.4238612833298));
#43765=CARTESIAN_POINT('',(22.9811689265378,-2.89756944144577,15.3));
#43766=CARTESIAN_POINT('Ctrl Pts',(22.877968161414,-2.77386128332979,15.4238612833298));
#43767=CARTESIAN_POINT('Ctrl Pts',(22.9293648449275,-2.83547118557317,15.3623442379097));
#43768=CARTESIAN_POINT('Ctrl Pts',(22.9811689265378,-2.89756944144577,15.3));
#43769=CARTESIAN_POINT('',(22.9811689265378,-2.89756944144577,11.2));
#43770=CARTESIAN_POINT('',(22.9811689265378,-2.89756944144577,11.));
#43771=CARTESIAN_POINT('',(22.8988337499022,-2.79887314750331,11.1011268524967));
#43772=CARTESIAN_POINT('Ctrl Pts',(22.9811689265378,-2.89756944144577,11.2));
#43773=CARTESIAN_POINT('Ctrl Pts',(22.9398717132847,-2.84806591130493,11.1503003777304));
#43774=CARTESIAN_POINT('Ctrl Pts',(22.8988337499022,-2.79887314750331,11.1011268524967));
#43775=CARTESIAN_POINT('',(22.8580624192708,-2.75,11.15));
#43776=CARTESIAN_POINT('',(22.0225261537486,-1.74843133601861,12.1515686639814));
#43777=CARTESIAN_POINT('',(22.8580624192708,-2.75,15.4));
#43778=CARTESIAN_POINT('',(22.8580624192708,-2.75,11.));
#43779=CARTESIAN_POINT('',(21.310816473291,-0.895295280514285,13.5452952805143));
#43780=CARTESIAN_POINT('Origin',(15.875,-2.8,15.45));
#43781=CARTESIAN_POINT('',(15.,-2.75,15.4));
#43782=CARTESIAN_POINT('',(15.875,-2.75,15.4));
#43783=CARTESIAN_POINT('',(15.,-2.85,15.5));
#43784=CARTESIAN_POINT('',(15.,-2.75,15.4));
#43785=CARTESIAN_POINT('',(22.6848608818125,-2.85,15.5));
#43786=CARTESIAN_POINT('',(15.875,-2.85,15.5));
#43787=CARTESIAN_POINT('',(22.8714720490513,-2.77928932188134,15.4292893218813));
#43788=CARTESIAN_POINT('Ctrl Pts',(22.8714720490514,-2.77928932188136,15.4292893218813));
#43789=CARTESIAN_POINT('Ctrl Pts',(22.8092954963184,-2.80289320050232,15.4528932005023));
#43790=CARTESIAN_POINT('Ctrl Pts',(22.7470894475605,-2.82646471883622,15.4764647188362));
#43791=CARTESIAN_POINT('Ctrl Pts',(22.6848608818126,-2.85000000000001,15.5));
#43792=CARTESIAN_POINT('Ctrl Pts',(22.8714720490513,-2.77928932188134,15.4292893218813));
#43793=CARTESIAN_POINT('Ctrl Pts',(22.8747201052327,-2.776575875968,15.426575875968));
#43794=CARTESIAN_POINT('Ctrl Pts',(22.877968161414,-2.77386128332979,15.4238612833298));
#43795=CARTESIAN_POINT('Origin',(24.25,-2.75,15.5));
#43796=CARTESIAN_POINT('',(15.,-2.75,11.15));
#43797=CARTESIAN_POINT('',(15.875,-2.75,11.15));
#43798=CARTESIAN_POINT('',(15.,-2.75,15.5));
#43799=CARTESIAN_POINT('Origin',(15.875,-2.825,11.075));
#43800=CARTESIAN_POINT('Ctrl Pts',(22.8988337499022,-2.79887314750332,11.1011268524967));
#43801=CARTESIAN_POINT('Ctrl Pts',(22.8380113137205,-2.84963708154272,11.0503629184573));
#43802=CARTESIAN_POINT('Ctrl Pts',(22.777188877539,-2.9,11.));
#43803=CARTESIAN_POINT('',(15.,-2.75,11.15));
#43804=CARTESIAN_POINT('Origin',(22.9196156729043,2.82378472072289,11.));
#43805=CARTESIAN_POINT('',(22.8580624192708,2.75,15.4));
#43806=CARTESIAN_POINT('',(20.7138618022943,0.179717612662962,12.8297176126629));
#43807=CARTESIAN_POINT('',(22.8580624192708,2.75,11.15));
#43808=CARTESIAN_POINT('',(22.8580624192708,2.75,11.));
#43809=CARTESIAN_POINT('',(21.4255714827519,1.03285366816728,12.8671463318327));
#43810=CARTESIAN_POINT('Origin',(11.25,2.825,11.075));
#43811=CARTESIAN_POINT('',(15.,2.75,11.15));
#43812=CARTESIAN_POINT('',(11.25,2.75,11.15));
#43813=CARTESIAN_POINT('',(15.,2.75,11.15));
#43814=CARTESIAN_POINT('Origin',(15.,0.,11.075));
#43815=CARTESIAN_POINT('Origin',(15.,0.,11.15));
#43816=CARTESIAN_POINT('Origin',(7.5,0.,11.1));
#43817=CARTESIAN_POINT('',(11.1460890181319,-15.3221582967889,11.2));
#43818=CARTESIAN_POINT('Origin',(7.5,0.,11.2));
#43819=CARTESIAN_POINT('',(11.0481336735778,-15.2443978869161,11.1018663264221));
#43820=CARTESIAN_POINT('Ctrl Pts',(11.0481336735779,-15.2443978869161,11.1018663264222));
#43821=CARTESIAN_POINT('Ctrl Pts',(11.0969582861968,-15.2831565876936,11.1506841026816));
#43822=CARTESIAN_POINT('Ctrl Pts',(11.1460890181319,-15.3221582967889,11.2));
#43823=CARTESIAN_POINT('Ctrl Pts',(11.15,-15.1155549021529,11.));
#43824=CARTESIAN_POINT('Ctrl Pts',(11.0992829893245,-15.1799763945344,11.0507170106755));
#43825=CARTESIAN_POINT('Ctrl Pts',(11.0481336735778,-15.2443978869161,11.1018663264221));
#43826=CARTESIAN_POINT('Origin',(15.,0.,15.5));
#43827=CARTESIAN_POINT('',(15.,2.75,15.4));
#43828=CARTESIAN_POINT('',(15.,2.75,15.5));
#43829=CARTESIAN_POINT('Origin',(15.,0.,15.4));
#43830=CARTESIAN_POINT('Origin',(15.,2.75,15.5));
#43831=CARTESIAN_POINT('',(11.25,2.75,15.4));
#43832=CARTESIAN_POINT('Origin',(7.5,0.,11.075));
#43833=CARTESIAN_POINT('',(5.495,-2.45541683229044E-16,11.15));
#43834=CARTESIAN_POINT('',(5.42,2.54726534222649E-16,11.075));
#43835=CARTESIAN_POINT('Origin',(7.5,0.,11.15));
#43836=CARTESIAN_POINT('Origin',(7.5,0.,15.5));
#43837=CARTESIAN_POINT('',(5.495,2.45541683229044E-16,15.4));
#43838=CARTESIAN_POINT('Origin',(7.5,0.,15.4));
#43839=CARTESIAN_POINT('',(5.495,2.45541683229044E-16,15.5));
#43840=CARTESIAN_POINT('Origin',(-8.03762184672835,2.0743466612552,11.));
#43841=CARTESIAN_POINT('',(-7.99388777632041,2.02441760835096,15.424417608351));
#43842=CARTESIAN_POINT('',(-8.10274389348871,2.1486933225104,15.3));
#43843=CARTESIAN_POINT('Ctrl Pts',(-7.99388777632041,2.02441760835096,15.424417608351));
#43844=CARTESIAN_POINT('Ctrl Pts',(-8.04810000436536,2.08630906224183,15.3626437619559));
#43845=CARTESIAN_POINT('Ctrl Pts',(-8.10274389348871,2.1486933225104,15.3));
#43846=CARTESIAN_POINT('',(-8.10274389348871,2.1486933225104,11.2));
#43847=CARTESIAN_POINT('',(-8.10274389348871,2.1486933225104,11.));
#43848=CARTESIAN_POINT('',(-8.01579995129907,2.04943366867993,11.1005663313201));
#43849=CARTESIAN_POINT('Ctrl Pts',(-8.10274389348871,2.1486933225104,11.2));
#43850=CARTESIAN_POINT('Ctrl Pts',(-8.05913426317107,2.09890633678157,11.1500059138463));
#43851=CARTESIAN_POINT('Ctrl Pts',(-8.01579995129907,2.04943366867993,11.1005663313201));
#43852=CARTESIAN_POINT('',(-7.97249979996799,2.,11.15));
#43853=CARTESIAN_POINT('',(-7.05685105019854,0.954648528195632,12.1953514718044));
#43854=CARTESIAN_POINT('',(-7.97249979996799,2.,15.4));
#43855=CARTESIAN_POINT('',(-7.97249979996799,2.,11.));
#43856=CARTESIAN_POINT('',(-6.32882477728353,0.12349647770076,13.5234964777007));
#43857=CARTESIAN_POINT('Origin',(-0.875,2.05,15.45));
#43858=CARTESIAN_POINT('',(1.15599253443404E-15,2.,15.4));
#43859=CARTESIAN_POINT('',(-0.875,2.,15.4));
#43860=CARTESIAN_POINT('',(1.11022302462516E-15,2.1,15.5));
#43861=CARTESIAN_POINT('',(1.15599253443404E-15,2.,15.4));
#43862=CARTESIAN_POINT('',(-7.80661621652545,2.1,15.5));
#43863=CARTESIAN_POINT('',(-0.875,2.1,15.5));
#43864=CARTESIAN_POINT('',(-7.9883371262892,2.02928932188135,15.4292893218813));
#43865=CARTESIAN_POINT('Ctrl Pts',(-7.9883371262892,2.02928932188135,15.4292893218813));
#43866=CARTESIAN_POINT('Ctrl Pts',(-7.92778701650562,2.05288762137753,15.4528876213775));
#43867=CARTESIAN_POINT('Ctrl Pts',(-7.86721103212806,2.07645911131076,15.4764591113107));
#43868=CARTESIAN_POINT('Ctrl Pts',(-7.80661621652544,2.1,15.5));
#43869=CARTESIAN_POINT('Ctrl Pts',(-7.9883371262892,2.02928932188135,15.4292893218813));
#43870=CARTESIAN_POINT('Ctrl Pts',(-7.99111245130481,2.02685390151439,15.4268539015144));
#43871=CARTESIAN_POINT('Ctrl Pts',(-7.99388777632041,2.02441760835096,15.424417608351));
#43872=CARTESIAN_POINT('Origin',(-9.25,2.,15.5));
#43873=CARTESIAN_POINT('',(1.15599253443404E-15,2.,11.15));
#43874=CARTESIAN_POINT('',(-0.875,2.,11.15));
#43875=CARTESIAN_POINT('',(1.15599253443404E-15,2.,15.5));
#43876=CARTESIAN_POINT('Origin',(-0.875,2.075,11.075));
#43877=CARTESIAN_POINT('Ctrl Pts',(-8.01579995129907,2.04943366867993,11.1005663313201));
#43878=CARTESIAN_POINT('Ctrl Pts',(-7.95822464412934,2.09990411772965,11.0500958822704));
#43879=CARTESIAN_POINT('Ctrl Pts',(-7.90064933695979,2.15,11.));
#43880=CARTESIAN_POINT('',(1.15599253443404E-15,2.,11.15));
#43881=CARTESIAN_POINT('Origin',(-8.03762184672835,-2.0743466612552,11.));
#43882=CARTESIAN_POINT('',(-8.01579995129907,-2.04943366867993,11.1005663313201));
#43883=CARTESIAN_POINT('',(-8.10274389348871,-2.14869332251039,11.2));
#43884=CARTESIAN_POINT('Ctrl Pts',(-8.01579995129907,-2.04943366867993,
11.1005663313201));
#43885=CARTESIAN_POINT('Ctrl Pts',(-8.05913426317095,-2.09890633678143,
11.1500059138462));
#43886=CARTESIAN_POINT('Ctrl Pts',(-8.10274389348871,-2.1486933225104,11.2));
#43887=CARTESIAN_POINT('',(-8.10274389348871,-2.14869332251039,15.3));
#43888=CARTESIAN_POINT('',(-8.10274389348871,-2.14869332251039,11.));
#43889=CARTESIAN_POINT('',(-7.99388777632041,-2.02441760835096,15.424417608351));
#43890=CARTESIAN_POINT('Ctrl Pts',(-8.10274389348871,-2.1486933225104,15.3));
#43891=CARTESIAN_POINT('Ctrl Pts',(-8.04810000436667,-2.08630906224331,
15.3626437619544));
#43892=CARTESIAN_POINT('Ctrl Pts',(-7.99388777632041,-2.02441760835096,
15.424417608351));
#43893=CARTESIAN_POINT('',(-7.97249979996799,-2.,15.4));
#43894=CARTESIAN_POINT('',(-5.68766313969174,0.608486459740959,12.791513540259));
#43895=CARTESIAN_POINT('',(-7.97249979996799,-2.,11.15));
#43896=CARTESIAN_POINT('',(-7.97249979996799,-2.,11.));
#43897=CARTESIAN_POINT('',(-6.41568941260673,-0.222665590753897,12.9273344092461));
#43898=CARTESIAN_POINT('Origin',(7.5,0.,11.));
#43899=CARTESIAN_POINT('',(3.85391098186813,-15.3221582967889,11.2));
#43900=CARTESIAN_POINT('Origin',(7.5,0.,11.2));
#43901=CARTESIAN_POINT('',(3.85391098186813,-15.3221582967889,15.3));
#43902=CARTESIAN_POINT('',(3.85391098186813,-15.3221582967889,11.));
#43903=CARTESIAN_POINT('Origin',(7.5,0.,15.3));
#43904=CARTESIAN_POINT('Origin',(7.5,0.,11.1));
#43905=CARTESIAN_POINT('Ctrl Pts',(-7.90064933695979,-2.15,11.));
#43906=CARTESIAN_POINT('Ctrl Pts',(-7.95822464412947,-2.09990411772952,
11.0500958822705));
#43907=CARTESIAN_POINT('Ctrl Pts',(-8.01579995129907,-2.04943366867993,
11.1005663313201));
#43908=CARTESIAN_POINT('',(3.95186632642215,-15.2443978869161,11.1018663264222));
#43909=CARTESIAN_POINT('Ctrl Pts',(3.95186632642215,-15.2443978869161,11.1018663264222));
#43910=CARTESIAN_POINT('Ctrl Pts',(3.90071701067554,-15.1799763945344,11.0507170106755));
#43911=CARTESIAN_POINT('Ctrl Pts',(3.85,-15.1155549021529,11.));
#43912=CARTESIAN_POINT('Ctrl Pts',(3.85391098186813,-15.3221582967889,11.2));
#43913=CARTESIAN_POINT('Ctrl Pts',(3.90304171380303,-15.2831565876938,11.1506841026818));
#43914=CARTESIAN_POINT('Ctrl Pts',(3.95186632642215,-15.2443978869161,11.1018663264222));
#43915=CARTESIAN_POINT('Origin',(3.75,-2.075,11.075));
#43916=CARTESIAN_POINT('',(-2.44929359829471E-16,-2.,11.15));
#43917=CARTESIAN_POINT('',(3.75,-2.,11.15));
#43918=CARTESIAN_POINT('',(-2.44929359829471E-16,-2.,11.15));
#43919=CARTESIAN_POINT('Origin',(3.33066907387547E-16,1.11022302462516E-15,
11.075));
#43920=CARTESIAN_POINT('Origin',(3.33066907387547E-16,1.11022302462516E-15,
11.15));
#43921=CARTESIAN_POINT('Origin',(3.33066907387547E-16,1.11022302462516E-15,
15.5));
#43922=CARTESIAN_POINT('',(-2.44929359829471E-16,-2.,15.4));
#43923=CARTESIAN_POINT('',(-2.44929359829471E-16,-2.,15.5));
#43924=CARTESIAN_POINT('Origin',(3.33066907387547E-16,1.11022302462516E-15,
15.4));
#43925=CARTESIAN_POINT('Origin',(-2.44929359829471E-16,-2.,15.5));
#43926=CARTESIAN_POINT('',(3.75,-2.,15.4));
#43927=CARTESIAN_POINT('Origin',(3.92695549093406,-15.2641729873626,11.));
#43928=CARTESIAN_POINT('',(3.9768743850762,-15.2245456072889,15.4231256149238));
#43929=CARTESIAN_POINT('Ctrl Pts',(3.9768743850762,-15.2245456072889,15.4231256149238));
#43930=CARTESIAN_POINT('Ctrl Pts',(3.91563394307748,-15.2731604316489,15.3619555845659));
#43931=CARTESIAN_POINT('Ctrl Pts',(3.85391098186813,-15.3221582967889,15.3));
#43932=CARTESIAN_POINT('',(4.,-15.2061876779362,11.15));
#43933=CARTESIAN_POINT('',(4.95122255935958,-14.4510736366054,12.1012225593596));
#43934=CARTESIAN_POINT('',(4.,-15.2061876779362,15.4));
#43935=CARTESIAN_POINT('',(4.,-15.2061876779362,11.));
#43936=CARTESIAN_POINT('',(5.82568926143346,-13.756891103911,13.5743107385665));
#43937=CARTESIAN_POINT('Origin',(3.95,-8.375,15.45));
#43938=CARTESIAN_POINT('',(4.,-7.5,15.4));
#43939=CARTESIAN_POINT('',(4.,-8.375,15.4));
#43940=CARTESIAN_POINT('',(3.9,-7.5,15.5));
#43941=CARTESIAN_POINT('',(4.,-7.5,15.4));
#43942=CARTESIAN_POINT('',(3.9,-15.0247296148716,15.5));
#43943=CARTESIAN_POINT('',(3.9,-8.375,15.5));
#43944=CARTESIAN_POINT('',(3.97071067811865,-15.2167906922565,15.4292893218813));
#43945=CARTESIAN_POINT('Ctrl Pts',(3.97071067811864,-15.2167906922566,15.4292893218815));
#43946=CARTESIAN_POINT('Ctrl Pts',(3.94710042961717,-15.152801460133,15.452899570383));
#43947=CARTESIAN_POINT('Ctrl Pts',(3.92352887530507,-15.08877879261,15.4764711246951));
#43948=CARTESIAN_POINT('Ctrl Pts',(3.89999999999998,-15.0247296148717,15.5000000000002));
#43949=CARTESIAN_POINT('Ctrl Pts',(3.97071067811865,-15.2167906922565,15.4292893218813));
#43950=CARTESIAN_POINT('Ctrl Pts',(3.97379174649682,-15.2206681497727,15.4262082535032));
#43951=CARTESIAN_POINT('Ctrl Pts',(3.9768743850762,-15.2245456072889,15.4231256149238));
#43952=CARTESIAN_POINT('Origin',(4.,-16.75,15.5));
#43953=CARTESIAN_POINT('',(4.,-7.5,11.15));
#43954=CARTESIAN_POINT('',(4.,-8.375,11.15));
#43955=CARTESIAN_POINT('',(4.,-7.5,15.5));
#43956=CARTESIAN_POINT('Origin',(3.925,-8.375,11.075));
#43957=CARTESIAN_POINT('',(4.,-7.5,11.15));
#43958=CARTESIAN_POINT('Origin',(11.0730445090659,-15.2641729873626,11.));
#43959=CARTESIAN_POINT('',(11.1460890181319,-15.3221582967889,15.3));
#43960=CARTESIAN_POINT('',(11.1460890181319,-15.3221582967889,11.));
#43961=CARTESIAN_POINT('',(11.0231256149238,-15.2245456072889,15.4231256149238));
#43962=CARTESIAN_POINT('Ctrl Pts',(11.1460890181319,-15.3221582967889,15.3));
#43963=CARTESIAN_POINT('Ctrl Pts',(11.084366056921,-15.2731604316477,15.3619555845674));
#43964=CARTESIAN_POINT('Ctrl Pts',(11.0231256149238,-15.2245456072889,15.4231256149238));
#43965=CARTESIAN_POINT('',(11.,-15.2061876779362,15.4));
#43966=CARTESIAN_POINT('',(8.47635547471623,-13.2028295809074,12.8763554747162));
#43967=CARTESIAN_POINT('',(11.,-15.2061876779362,11.15));
#43968=CARTESIAN_POINT('',(11.,-15.2061876779362,11.));
#43969=CARTESIAN_POINT('',(9.35082217679008,-13.8970121136018,12.7991778232099));
#43970=CARTESIAN_POINT('Origin',(7.5,0.,11.));
#43971=CARTESIAN_POINT('Origin',(7.5,0.,15.3));
#43972=CARTESIAN_POINT('Origin',(11.075,-3.75,11.075));
#43973=CARTESIAN_POINT('',(11.,-7.5,11.15));
#43974=CARTESIAN_POINT('',(11.,-3.75,11.15));
#43975=CARTESIAN_POINT('',(11.,-7.5,11.15));
#43976=CARTESIAN_POINT('Origin',(7.5,-7.5,11.075));
#43977=CARTESIAN_POINT('Origin',(7.5,-7.5,11.15));
#43978=CARTESIAN_POINT('Origin',(7.5,-7.5,15.5));
#43979=CARTESIAN_POINT('',(11.,-7.5,15.4));
#43980=CARTESIAN_POINT('',(11.,-7.5,15.5));
#43981=CARTESIAN_POINT('Origin',(7.5,-7.5,15.4));
#43982=CARTESIAN_POINT('Origin',(11.,-7.5,15.5));
#43983=CARTESIAN_POINT('',(11.,-3.75,15.4));
#43984=CARTESIAN_POINT('Origin',(7.5,-4.78246333309122E-16,15.4646446609407));
#43985=CARTESIAN_POINT('Origin',(7.5,0.,15.5));
#43986=CARTESIAN_POINT('Origin',(7.5,-9.56492666618245E-16,15.4292893218813));
#43987=CARTESIAN_POINT('Origin',(7.5,-4.78246333309122E-16,15.4646446609407));
#43988=CARTESIAN_POINT('',(-7.9883371262892,-2.02928932188134,15.4292893218813));
#43989=CARTESIAN_POINT('Origin',(7.5,-9.56492666618245E-16,15.4292893218813));
#43990=CARTESIAN_POINT('',(-7.80661621652546,-2.1,15.5));
#43991=CARTESIAN_POINT('Origin',(7.5,0.,15.5));
#43992=CARTESIAN_POINT('Ctrl Pts',(-7.80661621652547,-2.1,15.5));
#43993=CARTESIAN_POINT('Ctrl Pts',(-7.86721103212863,-2.07645911131055,
15.4764591113106));
#43994=CARTESIAN_POINT('Ctrl Pts',(-7.92778701650677,-2.05288762137709,
15.4528876213771));
#43995=CARTESIAN_POINT('Ctrl Pts',(-7.98833712628922,-2.02928932188135,
15.4292893218814));
#43996=CARTESIAN_POINT('Origin',(7.5,-4.78246333309122E-16,15.4646446609407));
#43997=CARTESIAN_POINT('',(22.6848608818125,2.85,15.5));
#43998=CARTESIAN_POINT('Origin',(7.5,0.,15.5));
#43999=CARTESIAN_POINT('Ctrl Pts',(22.6848608818124,2.84999999999997,15.5));
#44000=CARTESIAN_POINT('Ctrl Pts',(22.7470894475593,2.82646471883652,15.4764647188366));
#44001=CARTESIAN_POINT('Ctrl Pts',(22.8092954963163,2.80289320050296,15.452893200503));
#44002=CARTESIAN_POINT('Ctrl Pts',(22.8714720490512,2.77928932188132,15.4292893218814));
#44003=CARTESIAN_POINT('Origin',(7.5,-4.78246333309122E-16,15.4646446609407));
#44004=CARTESIAN_POINT('',(11.0292893218813,-15.2167906922565,15.4292893218813));
#44005=CARTESIAN_POINT('Origin',(7.5,-9.56492666618245E-16,15.4292893218813));
#44006=CARTESIAN_POINT('',(11.1,-15.0247296148716,15.5));
#44007=CARTESIAN_POINT('Origin',(7.5,0.,15.5));
#44008=CARTESIAN_POINT('Ctrl Pts',(11.1,-15.0247296148717,15.5000000000002));
#44009=CARTESIAN_POINT('Ctrl Pts',(11.0764711246955,-15.0887787926085,15.4764711246956));
#44010=CARTESIAN_POINT('Ctrl Pts',(11.0528995703839,-15.15280146013,15.4528995703841));
#44011=CARTESIAN_POINT('Ctrl Pts',(11.0292893218814,-15.2167906922566,15.4292893218815));
#44012=CARTESIAN_POINT('Origin',(15.,0.,15.45));
#44013=CARTESIAN_POINT('',(15.,2.85,15.5));
#44014=CARTESIAN_POINT('',(15.,2.75,15.4));
#44015=CARTESIAN_POINT('Origin',(15.,0.,15.5));
#44016=CARTESIAN_POINT('Origin',(11.25,2.8,15.45));
#44017=CARTESIAN_POINT('',(11.25,2.85,15.5));
#44018=CARTESIAN_POINT('Origin',(7.5,-7.5,15.45));
#44019=CARTESIAN_POINT('',(11.1,-7.5,15.5));
#44020=CARTESIAN_POINT('',(11.,-7.5,15.4));
#44021=CARTESIAN_POINT('Origin',(7.5,-7.5,15.5));
#44022=CARTESIAN_POINT('Origin',(11.05,-3.75,15.45));
#44023=CARTESIAN_POINT('Ctrl Pts',(11.0231256149238,-15.2245456072889,15.4231256149238));
#44024=CARTESIAN_POINT('Ctrl Pts',(11.0262082535032,-15.2206681497727,15.4262082535032));
#44025=CARTESIAN_POINT('Ctrl Pts',(11.0292893218813,-15.2167906922565,15.4292893218813));
#44026=CARTESIAN_POINT('',(11.1,-3.75,15.5));
#44027=CARTESIAN_POINT('Origin',(7.5,7.5,15.45));
#44028=CARTESIAN_POINT('Origin',(7.5,7.5,15.5));
#44029=CARTESIAN_POINT('Origin',(7.5,7.5,15.4));
#44030=CARTESIAN_POINT('Origin',(3.33066907387547E-16,1.11022302462516E-15,
15.45));
#44031=CARTESIAN_POINT('',(2.40522482451567E-16,-2.1,15.5));
#44032=CARTESIAN_POINT('',(-2.44929359829471E-16,-2.,15.4));
#44033=CARTESIAN_POINT('Origin',(3.33066907387547E-16,1.11022302462516E-15,
15.5));
#44034=CARTESIAN_POINT('Origin',(3.75,-2.05,15.45));
#44035=CARTESIAN_POINT('Ctrl Pts',(-7.99388777632041,-2.02441760835096,
15.424417608351));
#44036=CARTESIAN_POINT('Ctrl Pts',(-7.99111245130481,-2.0268539015144,15.4268539015144));
#44037=CARTESIAN_POINT('Ctrl Pts',(-7.9883371262892,-2.02928932188134,15.4292893218813));
#44038=CARTESIAN_POINT('',(3.75,-2.1,15.5));
#44039=CARTESIAN_POINT('Origin',(7.5,0.,15.4));
#44040=CARTESIAN_POINT('Origin',(7.5,0.,15.4));
#44041=CARTESIAN_POINT('Origin',(7.5,0.,15.5));
#44042=CARTESIAN_POINT('',(5.395,-2.57788151220518E-16,15.5));
#44043=CARTESIAN_POINT('Origin',(7.5,0.,15.5));
#44044=CARTESIAN_POINT('Origin',(7.5,0.,15.45));
#44045=CARTESIAN_POINT('',(5.445,-2.51664917224781E-16,15.45));
#44046=CARTESIAN_POINT('Origin',(7.5,7.5,15.5));
#44047=CARTESIAN_POINT('',(8.75,7.5,15.5));
#44048=CARTESIAN_POINT('Origin',(8.75,16.75,15.5));
#44049=CARTESIAN_POINT('Origin',(7.5,0.,15.4));
#44050=CARTESIAN_POINT('Origin',(7.5,0.,15.3));
#44051=CARTESIAN_POINT('Origin',(7.5,0.,11.));
#44052=CARTESIAN_POINT('Origin',(7.5,0.,11.2));
#44053=CARTESIAN_POINT('Origin',(7.5,0.,11.1));
#70727=UNCERTAINTY_MEASURE_WITH_UNIT(LENGTH_MEASURE(0.001),#70758,
'DISTANCE_ACCURACY_VALUE',
'Maximum model space distance between geometric entities at asserted c
onnectivities');
#70740=UNCERTAINTY_MEASURE_WITH_UNIT(LENGTH_MEASURE(0.001),#70758,
'DISTANCE_ACCURACY_VALUE',
'Maximum model space distance between geometric entities at asserted c
onnectivities');
#70744=(
GEOMETRIC_REPRESENTATION_CONTEXT(3)
GLOBAL_UNCERTAINTY_ASSIGNED_CONTEXT((#70727))
GLOBAL_UNIT_ASSIGNED_CONTEXT((#70758,#70760,#70761))
REPRESENTATION_CONTEXT('','3D')
);
#70757=(
GEOMETRIC_REPRESENTATION_CONTEXT(3)
GLOBAL_UNCERTAINTY_ASSIGNED_CONTEXT((#70740))
GLOBAL_UNIT_ASSIGNED_CONTEXT((#70758,#70760,#70761))
REPRESENTATION_CONTEXT('','3D')
);
#70758=(
LENGTH_UNIT()
NAMED_UNIT(*)
SI_UNIT(.CENTI.,.METRE.)
);
#70760=(
NAMED_UNIT(*)
PLANE_ANGLE_UNIT()
SI_UNIT($,.RADIAN.)
);
#70761=(
NAMED_UNIT(*)
SI_UNIT($,.STERADIAN.)
SOLID_ANGLE_UNIT()
);
#70765=SHAPE_DEFINITION_REPRESENTATION(#70781,#70820);
#70781=PRODUCT_DEFINITION_SHAPE('',$,#70837);
#70820=SHAPE_REPRESENTATION('',(#27283),#70744);
#70833=PRODUCT_DEFINITION_CONTEXT('part definition',#70883,'design');
#70837=PRODUCT_DEFINITION('2026-10-19-02-55-33-757',
'08_Rotary_Anvil_Plate_D315x45_4-Slot',#70853,#70833);
#70853=PRODUCT_DEFINITION_FORMATION('',$,#70888);
#70883=APPLICATION_CONTEXT(
'Core Data for Automotive Mechanical Design Process');
#70884=PRODUCT_CONTEXT('part definition',#70883,'mechanical');
#70888=PRODUCT('2026-10-19-02-55-33-757',
'08_Rotary_Anvil_Plate_D315x45_4-Slot',$,(#70884));
#71027=COLOUR_RGB('Light Blue',0.38,0.62,0.78);
#71028=FILL_AREA_STYLE_COLOUR('',#71027);
#71029=FILL_AREA_STYLE('',(#71028));
#71030=SURFACE_STYLE_FILL_AREA(#71029);
#71031=SURFACE_SIDE_STYLE('',(#71030));
#71032=SURFACE_STYLE_USAGE(.BOTH.,#71031);
#71033=PRESENTATION_STYLE_ASSIGNMENT((#71032));
ENDSEC;
END-ISO-10303-21;
